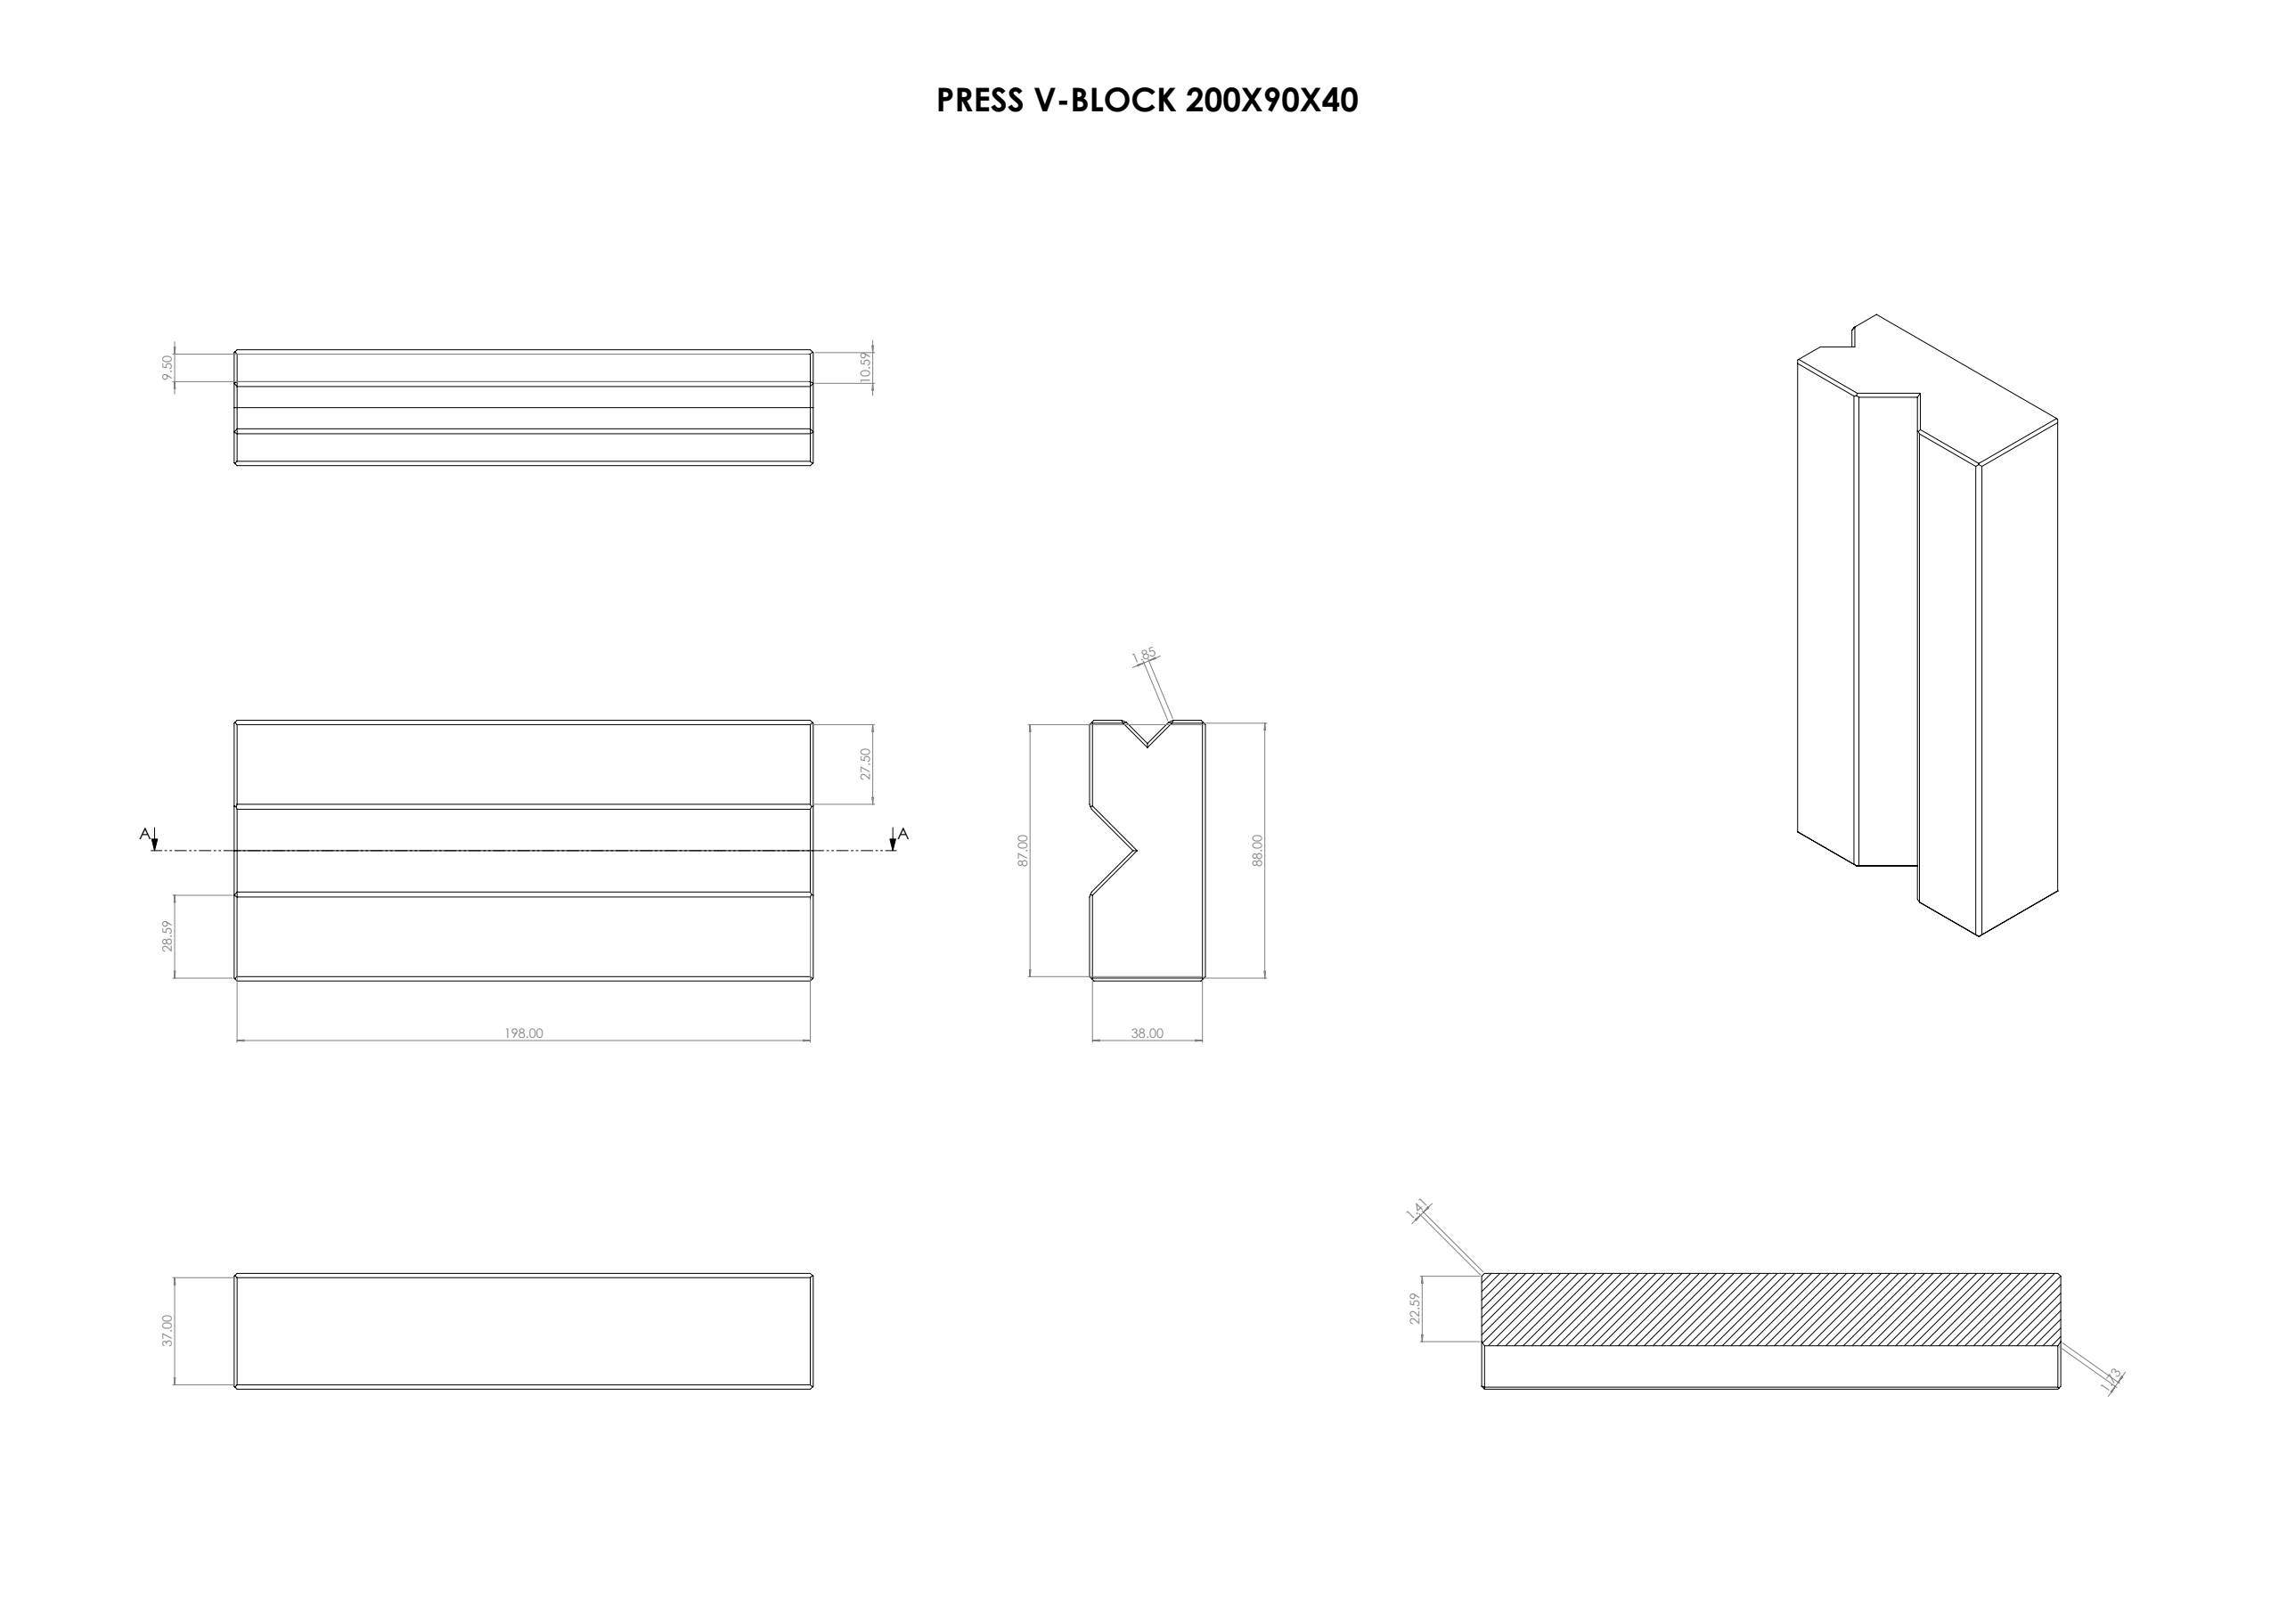
ISO-10303-21;
HEADER;
/* Generated by software containing ST-Developer
 * from STEP Tools, Inc. (www.steptools.com) 
 */

FILE_DESCRIPTION(
/* description */ (''),
/* implementation_level */ '2;1');

FILE_NAME(
/* name */ '16_Press_V-Block_200x90x40.step',
/* time_stamp */ '2026-10-20T10:03:03-07:00',
/* author */ (''),
/* organization */ (''),
/* preprocessor_version */ 'ST-DEVELOPER v20.2',
/* originating_system */ 'Autodesk Translation Framework v15.15.0.0',
/* authorisation */ '');

FILE_SCHEMA (('AUTOMOTIVE_DESIGN { 1 0 10303 214 3 1 1 }'));
ENDSEC;

DATA;
#10=MECHANICAL_DESIGN_GEOMETRIC_PRESENTATION_REPRESENTATION('',(#538),#71492);
#395=SHAPE_REPRESENTATION_RELATIONSHIP('SRR','None',#71616,#414);
#414=ADVANCED_BREP_SHAPE_REPRESENTATION('',(#433),#71486);
#433=MANIFOLD_SOLID_BREP('V-block',#28472);
#538=STYLED_ITEM('',(#71866),#433);
#4118=FACE_OUTER_BOUND('',#5800,.T.);
#4119=FACE_OUTER_BOUND('',#5801,.T.);
#4120=FACE_OUTER_BOUND('',#5802,.T.);
#4121=FACE_OUTER_BOUND('',#5803,.T.);
#4122=FACE_OUTER_BOUND('',#5804,.T.);
#4123=FACE_OUTER_BOUND('',#5805,.T.);
#4124=FACE_OUTER_BOUND('',#5806,.T.);
#4125=FACE_OUTER_BOUND('',#5807,.T.);
#4126=FACE_OUTER_BOUND('',#5808,.T.);
#4127=FACE_OUTER_BOUND('',#5809,.T.);
#4128=FACE_OUTER_BOUND('',#5810,.T.);
#4129=FACE_OUTER_BOUND('',#5811,.T.);
#4130=FACE_OUTER_BOUND('',#5812,.T.);
#4131=FACE_OUTER_BOUND('',#5813,.T.);
#4132=FACE_OUTER_BOUND('',#5814,.T.);
#4133=FACE_OUTER_BOUND('',#5815,.T.);
#4134=FACE_OUTER_BOUND('',#5816,.T.);
#4135=FACE_OUTER_BOUND('',#5817,.T.);
#4136=FACE_OUTER_BOUND('',#5818,.T.);
#4137=FACE_OUTER_BOUND('',#5819,.T.);
#4138=FACE_OUTER_BOUND('',#5820,.T.);
#4139=FACE_OUTER_BOUND('',#5821,.T.);
#4140=FACE_OUTER_BOUND('',#5822,.T.);
#4141=FACE_OUTER_BOUND('',#5823,.T.);
#4142=FACE_OUTER_BOUND('',#5824,.T.);
#4143=FACE_OUTER_BOUND('',#5825,.T.);
#4144=FACE_OUTER_BOUND('',#5826,.T.);
#4145=FACE_OUTER_BOUND('',#5827,.T.);
#4146=FACE_OUTER_BOUND('',#5828,.T.);
#4147=FACE_OUTER_BOUND('',#5829,.T.);
#4148=FACE_OUTER_BOUND('',#5830,.T.);
#4149=FACE_OUTER_BOUND('',#5831,.T.);
#4150=FACE_OUTER_BOUND('',#5832,.T.);
#4151=FACE_OUTER_BOUND('',#5833,.T.);
#4152=FACE_OUTER_BOUND('',#5834,.T.);
#4153=FACE_OUTER_BOUND('',#5835,.T.);
#4154=FACE_OUTER_BOUND('',#5836,.T.);
#4155=FACE_OUTER_BOUND('',#5837,.T.);
#4156=FACE_OUTER_BOUND('',#5838,.T.);
#4157=FACE_OUTER_BOUND('',#5839,.T.);
#4158=FACE_OUTER_BOUND('',#5840,.T.);
#4159=FACE_OUTER_BOUND('',#5841,.T.);
#4160=FACE_OUTER_BOUND('',#5842,.T.);
#4161=FACE_OUTER_BOUND('',#5843,.T.);
#4162=FACE_OUTER_BOUND('',#5844,.T.);
#5800=EDGE_LOOP('',(#23869,#23870,#23871,#23872,#23873,#23874));
#5801=EDGE_LOOP('',(#23875,#23876,#23877,#23878));
#5802=EDGE_LOOP('',(#23879,#23880,#23881,#23882,#23883,#23884));
#5803=EDGE_LOOP('',(#23885,#23886,#23887,#23888,#23889,#23890));
#5804=EDGE_LOOP('',(#23891,#23892,#23893,#23894,#23895,#23896,#23897,#23898,
#23899,#23900));
#5805=EDGE_LOOP('',(#23901,#23902,#23903,#23904));
#5806=EDGE_LOOP('',(#23905,#23906,#23907,#23908,#23909));
#5807=EDGE_LOOP('',(#23910,#23911,#23912,#23913,#23914,#23915));
#5808=EDGE_LOOP('',(#23916,#23917,#23918,#23919,#23920));
#5809=EDGE_LOOP('',(#23921,#23922,#23923,#23924,#23925,#23926));
#5810=EDGE_LOOP('',(#23927,#23928,#23929,#23930));
#5811=EDGE_LOOP('',(#23931,#23932,#23933,#23934,#23935,#23936));
#5812=EDGE_LOOP('',(#23937,#23938,#23939,#23940,#23941));
#5813=EDGE_LOOP('',(#23942,#23943,#23944,#23945));
#5814=EDGE_LOOP('',(#23946,#23947,#23948,#23949,#23950,#23951));
#5815=EDGE_LOOP('',(#23952,#23953,#23954,#23955,#23956,#23957));
#5816=EDGE_LOOP('',(#23958,#23959,#23960,#23961,#23962));
#5817=EDGE_LOOP('',(#23963,#23964,#23965));
#5818=EDGE_LOOP('',(#23966,#23967,#23968,#23969));
#5819=EDGE_LOOP('',(#23970,#23971,#23972,#23973,#23974));
#5820=EDGE_LOOP('',(#23975,#23976,#23977,#23978,#23979));
#5821=EDGE_LOOP('',(#23980,#23981,#23982,#23983));
#5822=EDGE_LOOP('',(#23984,#23985,#23986,#23987,#23988,#23989));
#5823=EDGE_LOOP('',(#23990,#23991,#23992,#23993,#23994,#23995));
#5824=EDGE_LOOP('',(#23996,#23997,#23998,#23999,#24000,#24001));
#5825=EDGE_LOOP('',(#24002,#24003,#24004,#24005,#24006));
#5826=EDGE_LOOP('',(#24007,#24008,#24009));
#5827=EDGE_LOOP('',(#24010,#24011,#24012,#24013,#24014));
#5828=EDGE_LOOP('',(#24015,#24016,#24017));
#5829=EDGE_LOOP('',(#24018,#24019,#24020,#24021));
#5830=EDGE_LOOP('',(#24022,#24023,#24024));
#5831=EDGE_LOOP('',(#24025,#24026,#24027,#24028));
#5832=EDGE_LOOP('',(#24029,#24030,#24031,#24032,#24033));
#5833=EDGE_LOOP('',(#24034,#24035,#24036));
#5834=EDGE_LOOP('',(#24037,#24038,#24039,#24040));
#5835=EDGE_LOOP('',(#24041,#24042,#24043,#24044));
#5836=EDGE_LOOP('',(#24045,#24046,#24047,#24048));
#5837=EDGE_LOOP('',(#24049,#24050,#24051,#24052));
#5838=EDGE_LOOP('',(#24053,#24054,#24055,#24056));
#5839=EDGE_LOOP('',(#24057,#24058,#24059,#24060,#24061,#24062,#24063,#24064,
#24065,#24066));
#5840=EDGE_LOOP('',(#24067,#24068,#24069,#24070));
#5841=EDGE_LOOP('',(#24071,#24072,#24073,#24074));
#5842=EDGE_LOOP('',(#24075,#24076,#24077,#24078));
#5843=EDGE_LOOP('',(#24079,#24080,#24081,#24082,#24083,#24084));
#5844=EDGE_LOOP('',(#24085,#24086,#24087,#24088));
#8268=LINE('',#58858,#10756);
#8269=LINE('',#58860,#10757);
#8270=LINE('',#58862,#10758);
#8271=LINE('',#58864,#10759);
#8272=LINE('',#58866,#10760);
#8273=LINE('',#58867,#10761);
#8274=LINE('',#58870,#10762);
#8275=LINE('',#58872,#10763);
#8276=LINE('',#58873,#10764);
#8277=LINE('',#58876,#10765);
#8278=LINE('',#58878,#10766);
#8279=LINE('',#58880,#10767);
#8280=LINE('',#58881,#10768);
#8281=LINE('',#58884,#10769);
#8282=LINE('',#58886,#10770);
#8283=LINE('',#58888,#10771);
#8284=LINE('',#58889,#10772);
#8285=LINE('',#58892,#10773);
#8286=LINE('',#58894,#10774);
#8287=LINE('',#58896,#10775);
#8288=LINE('',#58898,#10776);
#8289=LINE('',#58900,#10777);
#8290=LINE('',#58902,#10778);
#8291=LINE('',#58904,#10779);
#8292=LINE('',#58905,#10780);
#8293=LINE('',#58908,#10781);
#8294=LINE('',#58909,#10782);
#8295=LINE('',#58912,#10783);
#8296=LINE('',#58914,#10784);
#8297=LINE('',#58916,#10785);
#8298=LINE('',#58917,#10786);
#8299=LINE('',#58920,#10787);
#8300=LINE('',#58922,#10788);
#8301=LINE('',#58923,#10789);
#8302=LINE('',#58926,#10790);
#8303=LINE('',#58928,#10791);
#8304=LINE('',#58929,#10792);
#8305=LINE('',#58933,#10793);
#8306=LINE('',#58935,#10794);
#8307=LINE('',#58937,#10795);
#8308=LINE('',#58939,#10796);
#8309=LINE('',#58941,#10797);
#8310=LINE('',#58942,#10798);
#8311=LINE('',#58945,#10799);
#8312=LINE('',#58947,#10800);
#8313=LINE('',#58948,#10801);
#8314=LINE('',#58950,#10802);
#8315=LINE('',#58952,#10803);
#8316=LINE('',#58953,#10804);
#8317=LINE('',#58955,#10805);
#8318=LINE('',#58958,#10806);
#8319=LINE('',#58959,#10807);
#8320=LINE('',#58962,#10808);
#8321=LINE('',#58964,#10809);
#8322=LINE('',#58966,#10810);
#8323=LINE('',#58967,#10811);
#8324=LINE('',#58970,#10812);
#8325=LINE('',#58972,#10813);
#8326=LINE('',#58973,#10814);
#8327=LINE('',#58976,#10815);
#8328=LINE('',#58977,#10816);
#8329=LINE('',#58980,#10817);
#8330=LINE('',#58981,#10818);
#8331=LINE('',#58983,#10819);
#8332=LINE('',#58984,#10820);
#8333=LINE('',#58988,#10821);
#8334=LINE('',#58989,#10822);
#8335=LINE('',#58991,#10823);
#8336=LINE('',#58992,#10824);
#8337=LINE('',#58995,#10825);
#8338=LINE('',#58997,#10826);
#8339=LINE('',#58998,#10827);
#8340=LINE('',#59002,#10828);
#8341=LINE('',#59003,#10829);
#8342=LINE('',#59004,#10830);
#8343=LINE('',#59007,#10831);
#8344=LINE('',#59009,#10832);
#8345=LINE('',#59010,#10833);
#8346=LINE('',#59013,#10834);
#8347=LINE('',#59015,#10835);
#8348=LINE('',#59016,#10836);
#8349=LINE('',#59019,#10837);
#8350=LINE('',#59021,#10838);
#8351=LINE('',#59022,#10839);
#8352=LINE('',#59026,#10840);
#8353=LINE('',#59027,#10841);
#8354=LINE('',#59028,#10842);
#8355=LINE('',#59030,#10843);
#8356=LINE('',#59033,#10844);
#8357=LINE('',#59034,#10845);
#8358=LINE('',#59036,#10846);
#8359=LINE('',#59037,#10847);
#8360=LINE('',#59041,#10848);
#8361=LINE('',#59042,#10849);
#8362=LINE('',#59043,#10850);
#8363=LINE('',#59046,#10851);
#8364=LINE('',#59047,#10852);
#8365=LINE('',#59049,#10853);
#8366=LINE('',#59052,#10854);
#8367=LINE('',#59053,#10855);
#8368=LINE('',#59056,#10856);
#8369=LINE('',#59058,#10857);
#8370=LINE('',#59059,#10858);
#8371=LINE('',#59061,#10859);
#8372=LINE('',#59062,#10860);
#8373=LINE('',#59064,#10861);
#8374=LINE('',#59065,#10862);
#8375=LINE('',#59067,#10863);
#8376=LINE('',#59071,#10864);
#8377=LINE('',#59075,#10865);
#10756=VECTOR('',#35925,1.);
#10757=VECTOR('',#35926,1.);
#10758=VECTOR('',#35927,1.);
#10759=VECTOR('',#35928,1.);
#10760=VECTOR('',#35929,1.);
#10761=VECTOR('',#35930,1.);
#10762=VECTOR('',#35933,1.);
#10763=VECTOR('',#35934,1.);
#10764=VECTOR('',#35935,1.);
#10765=VECTOR('',#35938,1.);
#10766=VECTOR('',#35939,1.);
#10767=VECTOR('',#35940,1.);
#10768=VECTOR('',#35941,1.);
#10769=VECTOR('',#35944,1.);
#10770=VECTOR('',#35945,1.);
#10771=VECTOR('',#35946,1.);
#10772=VECTOR('',#35947,1.);
#10773=VECTOR('',#35950,1.);
#10774=VECTOR('',#35951,1.);
#10775=VECTOR('',#35952,1.);
#10776=VECTOR('',#35953,1.);
#10777=VECTOR('',#35954,1.);
#10778=VECTOR('',#35955,1.);
#10779=VECTOR('',#35956,1.);
#10780=VECTOR('',#35957,1.);
#10781=VECTOR('',#35960,1.);
#10782=VECTOR('',#35961,1.);
#10783=VECTOR('',#35964,1.);
#10784=VECTOR('',#35965,1.);
#10785=VECTOR('',#35966,1.);
#10786=VECTOR('',#35967,1.);
#10787=VECTOR('',#35970,1.);
#10788=VECTOR('',#35971,1.);
#10789=VECTOR('',#35972,1.);
#10790=VECTOR('',#35975,1.);
#10791=VECTOR('',#35976,1.);
#10792=VECTOR('',#35977,1.);
#10793=VECTOR('',#35980,1.);
#10794=VECTOR('',#35981,1.);
#10795=VECTOR('',#35982,1.);
#10796=VECTOR('',#35983,1.);
#10797=VECTOR('',#35984,1.);
#10798=VECTOR('',#35985,1.);
#10799=VECTOR('',#35988,1.);
#10800=VECTOR('',#35989,1.);
#10801=VECTOR('',#35990,1.);
#10802=VECTOR('',#35993,1.);
#10803=VECTOR('',#35994,1.);
#10804=VECTOR('',#35995,1.);
#10805=VECTOR('',#35998,1.);
#10806=VECTOR('',#36001,1.);
#10807=VECTOR('',#36002,1.);
#10808=VECTOR('',#36005,1.);
#10809=VECTOR('',#36006,1.);
#10810=VECTOR('',#36007,1.);
#10811=VECTOR('',#36008,1.);
#10812=VECTOR('',#36011,1.);
#10813=VECTOR('',#36012,1.);
#10814=VECTOR('',#36013,1.);
#10815=VECTOR('',#36016,1.);
#10816=VECTOR('',#36017,1.);
#10817=VECTOR('',#36020,1.);
#10818=VECTOR('',#36021,1.);
#10819=VECTOR('',#36024,1.);
#10820=VECTOR('',#36025,1.);
#10821=VECTOR('',#36028,1.);
#10822=VECTOR('',#36029,1.);
#10823=VECTOR('',#36030,1.);
#10824=VECTOR('',#36031,1.);
#10825=VECTOR('',#36034,1.);
#10826=VECTOR('',#36035,1.);
#10827=VECTOR('',#36036,1.);
#10828=VECTOR('',#36041,1.);
#10829=VECTOR('',#36042,1.);
#10830=VECTOR('',#36043,1.);
#10831=VECTOR('',#36046,1.);
#10832=VECTOR('',#36047,1.);
#10833=VECTOR('',#36048,1.);
#10834=VECTOR('',#36051,1.);
#10835=VECTOR('',#36052,1.);
#10836=VECTOR('',#36053,1.);
#10837=VECTOR('',#36056,1.);
#10838=VECTOR('',#36057,1.);
#10839=VECTOR('',#36058,1.);
#10840=VECTOR('',#36061,1.);
#10841=VECTOR('',#36062,1.);
#10842=VECTOR('',#36063,1.);
#10843=VECTOR('',#36066,1.);
#10844=VECTOR('',#36069,1.);
#10845=VECTOR('',#36070,1.);
#10846=VECTOR('',#36073,1.);
#10847=VECTOR('',#36074,1.);
#10848=VECTOR('',#36077,1.);
#10849=VECTOR('',#36078,1.);
#10850=VECTOR('',#36079,1.);
#10851=VECTOR('',#36082,1.);
#10852=VECTOR('',#36083,1.);
#10853=VECTOR('',#36086,1.);
#10854=VECTOR('',#36089,1.);
#10855=VECTOR('',#36090,1.);
#10856=VECTOR('',#36093,1.);
#10857=VECTOR('',#36094,1.);
#10858=VECTOR('',#36095,1.);
#10859=VECTOR('',#36098,1.);
#10860=VECTOR('',#36099,1.);
#10861=VECTOR('',#36102,1.);
#10862=VECTOR('',#36103,1.);
#10863=VECTOR('',#36106,1.);
#10864=VECTOR('',#36113,1.);
#10865=VECTOR('',#36120,1.);
#13146=VERTEX_POINT('',#58856);
#13147=VERTEX_POINT('',#58857);
#13148=VERTEX_POINT('',#58859);
#13149=VERTEX_POINT('',#58861);
#13150=VERTEX_POINT('',#58863);
#13151=VERTEX_POINT('',#58865);
#13152=VERTEX_POINT('',#58869);
#13153=VERTEX_POINT('',#58871);
#13154=VERTEX_POINT('',#58875);
#13155=VERTEX_POINT('',#58877);
#13156=VERTEX_POINT('',#58879);
#13157=VERTEX_POINT('',#58883);
#13158=VERTEX_POINT('',#58885);
#13159=VERTEX_POINT('',#58887);
#13160=VERTEX_POINT('',#58891);
#13161=VERTEX_POINT('',#58893);
#13162=VERTEX_POINT('',#58895);
#13163=VERTEX_POINT('',#58897);
#13164=VERTEX_POINT('',#58899);
#13165=VERTEX_POINT('',#58901);
#13166=VERTEX_POINT('',#58903);
#13167=VERTEX_POINT('',#58907);
#13168=VERTEX_POINT('',#58911);
#13169=VERTEX_POINT('',#58913);
#13170=VERTEX_POINT('',#58915);
#13171=VERTEX_POINT('',#58919);
#13172=VERTEX_POINT('',#58921);
#13173=VERTEX_POINT('',#58925);
#13174=VERTEX_POINT('',#58927);
#13175=VERTEX_POINT('',#58931);
#13176=VERTEX_POINT('',#58932);
#13177=VERTEX_POINT('',#58934);
#13178=VERTEX_POINT('',#58936);
#13179=VERTEX_POINT('',#58938);
#13180=VERTEX_POINT('',#58940);
#13181=VERTEX_POINT('',#58944);
#13182=VERTEX_POINT('',#58946);
#13183=VERTEX_POINT('',#58951);
#13184=VERTEX_POINT('',#58957);
#13185=VERTEX_POINT('',#58961);
#13186=VERTEX_POINT('',#58963);
#13187=VERTEX_POINT('',#58965);
#13188=VERTEX_POINT('',#58969);
#13189=VERTEX_POINT('',#58971);
#13190=VERTEX_POINT('',#58975);
#13191=VERTEX_POINT('',#58979);
#13192=VERTEX_POINT('',#58986);
#13193=VERTEX_POINT('',#58987);
#13194=VERTEX_POINT('',#58990);
#13195=VERTEX_POINT('',#58994);
#13196=VERTEX_POINT('',#58996);
#13197=VERTEX_POINT('',#59001);
#13198=VERTEX_POINT('',#59006);
#13199=VERTEX_POINT('',#59008);
#13200=VERTEX_POINT('',#59012);
#13201=VERTEX_POINT('',#59014);
#13202=VERTEX_POINT('',#59018);
#13203=VERTEX_POINT('',#59020);
#13204=VERTEX_POINT('',#59024);
#13205=VERTEX_POINT('',#59025);
#13206=VERTEX_POINT('',#59032);
#13207=VERTEX_POINT('',#59039);
#13208=VERTEX_POINT('',#59040);
#13209=VERTEX_POINT('',#59045);
#13210=VERTEX_POINT('',#59051);
#13211=VERTEX_POINT('',#59055);
#13212=VERTEX_POINT('',#59057);
#16818=EDGE_CURVE('',#13146,#13147,#8268,.T.);
#16819=EDGE_CURVE('',#13147,#13148,#8269,.T.);
#16820=EDGE_CURVE('',#13148,#13149,#8270,.T.);
#16821=EDGE_CURVE('',#13149,#13150,#8271,.T.);
#16822=EDGE_CURVE('',#13150,#13151,#8272,.T.);
#16823=EDGE_CURVE('',#13151,#13146,#8273,.T.);
#16824=EDGE_CURVE('',#13152,#13150,#8274,.T.);
#16825=EDGE_CURVE('',#13153,#13152,#8275,.T.);
#16826=EDGE_CURVE('',#13151,#13153,#8276,.T.);
#16827=EDGE_CURVE('',#13154,#13149,#8277,.T.);
#16828=EDGE_CURVE('',#13154,#13155,#8278,.T.);
#16829=EDGE_CURVE('',#13156,#13155,#8279,.T.);
#16830=EDGE_CURVE('',#13152,#13156,#8280,.T.);
#16831=EDGE_CURVE('',#13148,#13157,#8281,.T.);
#16832=EDGE_CURVE('',#13157,#13158,#8282,.T.);
#16833=EDGE_CURVE('',#13158,#13159,#8283,.T.);
#16834=EDGE_CURVE('',#13159,#13154,#8284,.T.);
#16835=EDGE_CURVE('',#13160,#13147,#8285,.T.);
#16836=EDGE_CURVE('',#13161,#13160,#8286,.T.);
#16837=EDGE_CURVE('',#13162,#13161,#8287,.T.);
#16838=EDGE_CURVE('',#13163,#13162,#8288,.T.);
#16839=EDGE_CURVE('',#13164,#13163,#8289,.T.);
#16840=EDGE_CURVE('',#13165,#13164,#8290,.T.);
#16841=EDGE_CURVE('',#13166,#13165,#8291,.T.);
#16842=EDGE_CURVE('',#13157,#13166,#8292,.T.);
#16843=EDGE_CURVE('',#13167,#13159,#8293,.T.);
#16844=EDGE_CURVE('',#13155,#13167,#8294,.T.);
#16845=EDGE_CURVE('',#13168,#13166,#8295,.T.);
#16846=EDGE_CURVE('',#13165,#13169,#8296,.F.);
#16847=EDGE_CURVE('',#13169,#13170,#8297,.T.);
#16848=EDGE_CURVE('',#13170,#13168,#8298,.T.);
#16849=EDGE_CURVE('',#13171,#13168,#8299,.T.);
#16850=EDGE_CURVE('',#13171,#13172,#8300,.T.);
#16851=EDGE_CURVE('',#13172,#13158,#8301,.T.);
#16852=EDGE_CURVE('',#13170,#13173,#8302,.T.);
#16853=EDGE_CURVE('',#13173,#13174,#8303,.T.);
#16854=EDGE_CURVE('',#13174,#13171,#8304,.T.);
#16855=EDGE_CURVE('',#13175,#13176,#8305,.T.);
#16856=EDGE_CURVE('',#13176,#13177,#8306,.T.);
#16857=EDGE_CURVE('',#13177,#13178,#8307,.T.);
#16858=EDGE_CURVE('',#13178,#13179,#8308,.T.);
#16859=EDGE_CURVE('',#13179,#13180,#8309,.T.);
#16860=EDGE_CURVE('',#13180,#13175,#8310,.T.);
#16861=EDGE_CURVE('',#13181,#13176,#8311,.T.);
#16862=EDGE_CURVE('',#13182,#13181,#8312,.T.);
#16863=EDGE_CURVE('',#13177,#13182,#8313,.T.);
#16864=EDGE_CURVE('',#13164,#13175,#8314,.T.);
#16865=EDGE_CURVE('',#13163,#13183,#8315,.T.);
#16866=EDGE_CURVE('',#13183,#13181,#8316,.T.);
#16867=EDGE_CURVE('',#13180,#13169,#8317,.T.);
#16868=EDGE_CURVE('',#13184,#13179,#8318,.T.);
#16869=EDGE_CURVE('',#13184,#13169,#8319,.T.);
#16870=EDGE_CURVE('',#13185,#13183,#8320,.T.);
#16871=EDGE_CURVE('',#13185,#13186,#8321,.T.);
#16872=EDGE_CURVE('',#13187,#13186,#8322,.T.);
#16873=EDGE_CURVE('',#13182,#13187,#8323,.T.);
#16874=EDGE_CURVE('',#13187,#13188,#8324,.T.);
#16875=EDGE_CURVE('',#13188,#13189,#8325,.T.);
#16876=EDGE_CURVE('',#13189,#13178,#8326,.T.);
#16877=EDGE_CURVE('',#13189,#13190,#8327,.T.);
#16878=EDGE_CURVE('',#13190,#13184,#8328,.T.);
#16879=EDGE_CURVE('',#13191,#13173,#8329,.T.);
#16880=EDGE_CURVE('',#13174,#13191,#8330,.T.);
#16881=EDGE_CURVE('',#13190,#13191,#8331,.T.);
#16882=EDGE_CURVE('',#13173,#13184,#8332,.T.);
#16883=EDGE_CURVE('',#13192,#13193,#8333,.T.);
#16884=EDGE_CURVE('',#13193,#13174,#8334,.T.);
#16885=EDGE_CURVE('',#13191,#13194,#8335,.T.);
#16886=EDGE_CURVE('',#13194,#13192,#8336,.T.);
#16887=EDGE_CURVE('',#13186,#13195,#8337,.T.);
#16888=EDGE_CURVE('',#13195,#13196,#8338,.T.);
#16889=EDGE_CURVE('',#13196,#13188,#8339,.T.);
#16890=EDGE_CURVE('',#13194,#13197,#8340,.T.);
#16891=EDGE_CURVE('',#13197,#13156,#8341,.T.);
#16892=EDGE_CURVE('',#13167,#13192,#8342,.T.);
#16893=EDGE_CURVE('',#13197,#13198,#8343,.T.);
#16894=EDGE_CURVE('',#13198,#13199,#8344,.T.);
#16895=EDGE_CURVE('',#13199,#13153,#8345,.T.);
#16896=EDGE_CURVE('',#13200,#13199,#8346,.T.);
#16897=EDGE_CURVE('',#13200,#13201,#8347,.T.);
#16898=EDGE_CURVE('',#13146,#13201,#8348,.T.);
#16899=EDGE_CURVE('',#13198,#13202,#8349,.T.);
#16900=EDGE_CURVE('',#13202,#13203,#8350,.T.);
#16901=EDGE_CURVE('',#13203,#13200,#8351,.T.);
#16902=EDGE_CURVE('',#13204,#13205,#8352,.T.);
#16903=EDGE_CURVE('',#13162,#13204,#8353,.T.);
#16904=EDGE_CURVE('',#13205,#13162,#8354,.T.);
#16905=EDGE_CURVE('',#13204,#13185,#8355,.T.);
#16906=EDGE_CURVE('',#13206,#13195,#8356,.T.);
#16907=EDGE_CURVE('',#13196,#13206,#8357,.T.);
#16908=EDGE_CURVE('',#13195,#13204,#8358,.T.);
#16909=EDGE_CURVE('',#13205,#13206,#8359,.T.);
#16910=EDGE_CURVE('',#13207,#13208,#8360,.T.);
#16911=EDGE_CURVE('',#13160,#13207,#8361,.T.);
#16912=EDGE_CURVE('',#13208,#13160,#8362,.T.);
#16913=EDGE_CURVE('',#13207,#13209,#8363,.T.);
#16914=EDGE_CURVE('',#13209,#13161,#8364,.T.);
#16915=EDGE_CURVE('',#13201,#13208,#8365,.T.);
#16916=EDGE_CURVE('',#13203,#13210,#8366,.T.);
#16917=EDGE_CURVE('',#13210,#13202,#8367,.T.);
#16918=EDGE_CURVE('',#13211,#13210,#8368,.T.);
#16919=EDGE_CURVE('',#13202,#13212,#8369,.T.);
#16920=EDGE_CURVE('',#13212,#13211,#8370,.T.);
#16921=EDGE_CURVE('',#13208,#13203,#8371,.T.);
#16922=EDGE_CURVE('',#13210,#13207,#8372,.T.);
#16923=EDGE_CURVE('',#13212,#13196,#8373,.T.);
#16924=EDGE_CURVE('',#13206,#13211,#8374,.T.);
#16925=EDGE_CURVE('',#13209,#13205,#8375,.T.);
#16926=EDGE_CURVE('',#13211,#13209,#8376,.T.);
#16927=EDGE_CURVE('',#13172,#13193,#8377,.T.);
#23869=ORIENTED_EDGE('',*,*,#16818,.T.);
#23870=ORIENTED_EDGE('',*,*,#16819,.T.);
#23871=ORIENTED_EDGE('',*,*,#16820,.T.);
#23872=ORIENTED_EDGE('',*,*,#16821,.T.);
#23873=ORIENTED_EDGE('',*,*,#16822,.T.);
#23874=ORIENTED_EDGE('',*,*,#16823,.T.);
#23875=ORIENTED_EDGE('',*,*,#16822,.F.);
#23876=ORIENTED_EDGE('',*,*,#16824,.F.);
#23877=ORIENTED_EDGE('',*,*,#16825,.F.);
#23878=ORIENTED_EDGE('',*,*,#16826,.F.);
#23879=ORIENTED_EDGE('',*,*,#16821,.F.);
#23880=ORIENTED_EDGE('',*,*,#16827,.F.);
#23881=ORIENTED_EDGE('',*,*,#16828,.T.);
#23882=ORIENTED_EDGE('',*,*,#16829,.F.);
#23883=ORIENTED_EDGE('',*,*,#16830,.F.);
#23884=ORIENTED_EDGE('',*,*,#16824,.T.);
#23885=ORIENTED_EDGE('',*,*,#16820,.F.);
#23886=ORIENTED_EDGE('',*,*,#16831,.T.);
#23887=ORIENTED_EDGE('',*,*,#16832,.T.);
#23888=ORIENTED_EDGE('',*,*,#16833,.T.);
#23889=ORIENTED_EDGE('',*,*,#16834,.T.);
#23890=ORIENTED_EDGE('',*,*,#16827,.T.);
#23891=ORIENTED_EDGE('',*,*,#16819,.F.);
#23892=ORIENTED_EDGE('',*,*,#16835,.F.);
#23893=ORIENTED_EDGE('',*,*,#16836,.F.);
#23894=ORIENTED_EDGE('',*,*,#16837,.F.);
#23895=ORIENTED_EDGE('',*,*,#16838,.F.);
#23896=ORIENTED_EDGE('',*,*,#16839,.F.);
#23897=ORIENTED_EDGE('',*,*,#16840,.F.);
#23898=ORIENTED_EDGE('',*,*,#16841,.F.);
#23899=ORIENTED_EDGE('',*,*,#16842,.F.);
#23900=ORIENTED_EDGE('',*,*,#16831,.F.);
#23901=ORIENTED_EDGE('',*,*,#16834,.F.);
#23902=ORIENTED_EDGE('',*,*,#16843,.F.);
#23903=ORIENTED_EDGE('',*,*,#16844,.F.);
#23904=ORIENTED_EDGE('',*,*,#16828,.F.);
#23905=ORIENTED_EDGE('',*,*,#16845,.T.);
#23906=ORIENTED_EDGE('',*,*,#16841,.T.);
#23907=ORIENTED_EDGE('',*,*,#16846,.T.);
#23908=ORIENTED_EDGE('',*,*,#16847,.T.);
#23909=ORIENTED_EDGE('',*,*,#16848,.T.);
#23910=ORIENTED_EDGE('',*,*,#16832,.F.);
#23911=ORIENTED_EDGE('',*,*,#16842,.T.);
#23912=ORIENTED_EDGE('',*,*,#16845,.F.);
#23913=ORIENTED_EDGE('',*,*,#16849,.F.);
#23914=ORIENTED_EDGE('',*,*,#16850,.T.);
#23915=ORIENTED_EDGE('',*,*,#16851,.T.);
#23916=ORIENTED_EDGE('',*,*,#16848,.F.);
#23917=ORIENTED_EDGE('',*,*,#16852,.T.);
#23918=ORIENTED_EDGE('',*,*,#16853,.T.);
#23919=ORIENTED_EDGE('',*,*,#16854,.T.);
#23920=ORIENTED_EDGE('',*,*,#16849,.T.);
#23921=ORIENTED_EDGE('',*,*,#16855,.T.);
#23922=ORIENTED_EDGE('',*,*,#16856,.T.);
#23923=ORIENTED_EDGE('',*,*,#16857,.T.);
#23924=ORIENTED_EDGE('',*,*,#16858,.T.);
#23925=ORIENTED_EDGE('',*,*,#16859,.T.);
#23926=ORIENTED_EDGE('',*,*,#16860,.T.);
#23927=ORIENTED_EDGE('',*,*,#16856,.F.);
#23928=ORIENTED_EDGE('',*,*,#16861,.F.);
#23929=ORIENTED_EDGE('',*,*,#16862,.F.);
#23930=ORIENTED_EDGE('',*,*,#16863,.F.);
#23931=ORIENTED_EDGE('',*,*,#16855,.F.);
#23932=ORIENTED_EDGE('',*,*,#16864,.F.);
#23933=ORIENTED_EDGE('',*,*,#16839,.T.);
#23934=ORIENTED_EDGE('',*,*,#16865,.T.);
#23935=ORIENTED_EDGE('',*,*,#16866,.T.);
#23936=ORIENTED_EDGE('',*,*,#16861,.T.);
#23937=ORIENTED_EDGE('',*,*,#16860,.F.);
#23938=ORIENTED_EDGE('',*,*,#16867,.T.);
#23939=ORIENTED_EDGE('',*,*,#16846,.F.);
#23940=ORIENTED_EDGE('',*,*,#16840,.T.);
#23941=ORIENTED_EDGE('',*,*,#16864,.T.);
#23942=ORIENTED_EDGE('',*,*,#16859,.F.);
#23943=ORIENTED_EDGE('',*,*,#16868,.F.);
#23944=ORIENTED_EDGE('',*,*,#16869,.T.);
#23945=ORIENTED_EDGE('',*,*,#16867,.F.);
#23946=ORIENTED_EDGE('',*,*,#16866,.F.);
#23947=ORIENTED_EDGE('',*,*,#16870,.F.);
#23948=ORIENTED_EDGE('',*,*,#16871,.T.);
#23949=ORIENTED_EDGE('',*,*,#16872,.F.);
#23950=ORIENTED_EDGE('',*,*,#16873,.F.);
#23951=ORIENTED_EDGE('',*,*,#16862,.T.);
#23952=ORIENTED_EDGE('',*,*,#16857,.F.);
#23953=ORIENTED_EDGE('',*,*,#16863,.T.);
#23954=ORIENTED_EDGE('',*,*,#16873,.T.);
#23955=ORIENTED_EDGE('',*,*,#16874,.T.);
#23956=ORIENTED_EDGE('',*,*,#16875,.T.);
#23957=ORIENTED_EDGE('',*,*,#16876,.T.);
#23958=ORIENTED_EDGE('',*,*,#16858,.F.);
#23959=ORIENTED_EDGE('',*,*,#16876,.F.);
#23960=ORIENTED_EDGE('',*,*,#16877,.T.);
#23961=ORIENTED_EDGE('',*,*,#16878,.T.);
#23962=ORIENTED_EDGE('',*,*,#16868,.T.);
#23963=ORIENTED_EDGE('',*,*,#16853,.F.);
#23964=ORIENTED_EDGE('',*,*,#16879,.F.);
#23965=ORIENTED_EDGE('',*,*,#16880,.F.);
#23966=ORIENTED_EDGE('',*,*,#16881,.T.);
#23967=ORIENTED_EDGE('',*,*,#16879,.T.);
#23968=ORIENTED_EDGE('',*,*,#16882,.T.);
#23969=ORIENTED_EDGE('',*,*,#16878,.F.);
#23970=ORIENTED_EDGE('',*,*,#16883,.T.);
#23971=ORIENTED_EDGE('',*,*,#16884,.T.);
#23972=ORIENTED_EDGE('',*,*,#16880,.T.);
#23973=ORIENTED_EDGE('',*,*,#16885,.T.);
#23974=ORIENTED_EDGE('',*,*,#16886,.T.);
#23975=ORIENTED_EDGE('',*,*,#16874,.F.);
#23976=ORIENTED_EDGE('',*,*,#16872,.T.);
#23977=ORIENTED_EDGE('',*,*,#16887,.T.);
#23978=ORIENTED_EDGE('',*,*,#16888,.T.);
#23979=ORIENTED_EDGE('',*,*,#16889,.T.);
#23980=ORIENTED_EDGE('',*,*,#16847,.F.);
#23981=ORIENTED_EDGE('',*,*,#16869,.F.);
#23982=ORIENTED_EDGE('',*,*,#16882,.F.);
#23983=ORIENTED_EDGE('',*,*,#16852,.F.);
#23984=ORIENTED_EDGE('',*,*,#16886,.F.);
#23985=ORIENTED_EDGE('',*,*,#16890,.T.);
#23986=ORIENTED_EDGE('',*,*,#16891,.T.);
#23987=ORIENTED_EDGE('',*,*,#16829,.T.);
#23988=ORIENTED_EDGE('',*,*,#16844,.T.);
#23989=ORIENTED_EDGE('',*,*,#16892,.T.);
#23990=ORIENTED_EDGE('',*,*,#16891,.F.);
#23991=ORIENTED_EDGE('',*,*,#16893,.T.);
#23992=ORIENTED_EDGE('',*,*,#16894,.T.);
#23993=ORIENTED_EDGE('',*,*,#16895,.T.);
#23994=ORIENTED_EDGE('',*,*,#16825,.T.);
#23995=ORIENTED_EDGE('',*,*,#16830,.T.);
#23996=ORIENTED_EDGE('',*,*,#16823,.F.);
#23997=ORIENTED_EDGE('',*,*,#16826,.T.);
#23998=ORIENTED_EDGE('',*,*,#16895,.F.);
#23999=ORIENTED_EDGE('',*,*,#16896,.F.);
#24000=ORIENTED_EDGE('',*,*,#16897,.T.);
#24001=ORIENTED_EDGE('',*,*,#16898,.F.);
#24002=ORIENTED_EDGE('',*,*,#16894,.F.);
#24003=ORIENTED_EDGE('',*,*,#16899,.T.);
#24004=ORIENTED_EDGE('',*,*,#16900,.T.);
#24005=ORIENTED_EDGE('',*,*,#16901,.T.);
#24006=ORIENTED_EDGE('',*,*,#16896,.T.);
#24007=ORIENTED_EDGE('',*,*,#16902,.F.);
#24008=ORIENTED_EDGE('',*,*,#16903,.F.);
#24009=ORIENTED_EDGE('',*,*,#16904,.F.);
#24010=ORIENTED_EDGE('',*,*,#16865,.F.);
#24011=ORIENTED_EDGE('',*,*,#16838,.T.);
#24012=ORIENTED_EDGE('',*,*,#16903,.T.);
#24013=ORIENTED_EDGE('',*,*,#16905,.T.);
#24014=ORIENTED_EDGE('',*,*,#16870,.T.);
#24015=ORIENTED_EDGE('',*,*,#16888,.F.);
#24016=ORIENTED_EDGE('',*,*,#16906,.F.);
#24017=ORIENTED_EDGE('',*,*,#16907,.F.);
#24018=ORIENTED_EDGE('',*,*,#16906,.T.);
#24019=ORIENTED_EDGE('',*,*,#16908,.T.);
#24020=ORIENTED_EDGE('',*,*,#16902,.T.);
#24021=ORIENTED_EDGE('',*,*,#16909,.T.);
#24022=ORIENTED_EDGE('',*,*,#16910,.F.);
#24023=ORIENTED_EDGE('',*,*,#16911,.F.);
#24024=ORIENTED_EDGE('',*,*,#16912,.F.);
#24025=ORIENTED_EDGE('',*,*,#16836,.T.);
#24026=ORIENTED_EDGE('',*,*,#16911,.T.);
#24027=ORIENTED_EDGE('',*,*,#16913,.T.);
#24028=ORIENTED_EDGE('',*,*,#16914,.T.);
#24029=ORIENTED_EDGE('',*,*,#16818,.F.);
#24030=ORIENTED_EDGE('',*,*,#16898,.T.);
#24031=ORIENTED_EDGE('',*,*,#16915,.T.);
#24032=ORIENTED_EDGE('',*,*,#16912,.T.);
#24033=ORIENTED_EDGE('',*,*,#16835,.T.);
#24034=ORIENTED_EDGE('',*,*,#16916,.F.);
#24035=ORIENTED_EDGE('',*,*,#16900,.F.);
#24036=ORIENTED_EDGE('',*,*,#16917,.F.);
#24037=ORIENTED_EDGE('',*,*,#16918,.T.);
#24038=ORIENTED_EDGE('',*,*,#16917,.T.);
#24039=ORIENTED_EDGE('',*,*,#16919,.T.);
#24040=ORIENTED_EDGE('',*,*,#16920,.T.);
#24041=ORIENTED_EDGE('',*,*,#16910,.T.);
#24042=ORIENTED_EDGE('',*,*,#16921,.T.);
#24043=ORIENTED_EDGE('',*,*,#16916,.T.);
#24044=ORIENTED_EDGE('',*,*,#16922,.T.);
#24045=ORIENTED_EDGE('',*,*,#16923,.T.);
#24046=ORIENTED_EDGE('',*,*,#16907,.T.);
#24047=ORIENTED_EDGE('',*,*,#16924,.T.);
#24048=ORIENTED_EDGE('',*,*,#16920,.F.);
#24049=ORIENTED_EDGE('',*,*,#16925,.T.);
#24050=ORIENTED_EDGE('',*,*,#16904,.T.);
#24051=ORIENTED_EDGE('',*,*,#16837,.T.);
#24052=ORIENTED_EDGE('',*,*,#16914,.F.);
#24053=ORIENTED_EDGE('',*,*,#16905,.F.);
#24054=ORIENTED_EDGE('',*,*,#16908,.F.);
#24055=ORIENTED_EDGE('',*,*,#16887,.F.);
#24056=ORIENTED_EDGE('',*,*,#16871,.F.);
#24057=ORIENTED_EDGE('',*,*,#16875,.F.);
#24058=ORIENTED_EDGE('',*,*,#16889,.F.);
#24059=ORIENTED_EDGE('',*,*,#16923,.F.);
#24060=ORIENTED_EDGE('',*,*,#16919,.F.);
#24061=ORIENTED_EDGE('',*,*,#16899,.F.);
#24062=ORIENTED_EDGE('',*,*,#16893,.F.);
#24063=ORIENTED_EDGE('',*,*,#16890,.F.);
#24064=ORIENTED_EDGE('',*,*,#16885,.F.);
#24065=ORIENTED_EDGE('',*,*,#16881,.F.);
#24066=ORIENTED_EDGE('',*,*,#16877,.F.);
#24067=ORIENTED_EDGE('',*,*,#16913,.F.);
#24068=ORIENTED_EDGE('',*,*,#16922,.F.);
#24069=ORIENTED_EDGE('',*,*,#16918,.F.);
#24070=ORIENTED_EDGE('',*,*,#16926,.T.);
#24071=ORIENTED_EDGE('',*,*,#16925,.F.);
#24072=ORIENTED_EDGE('',*,*,#16926,.F.);
#24073=ORIENTED_EDGE('',*,*,#16924,.F.);
#24074=ORIENTED_EDGE('',*,*,#16909,.F.);
#24075=ORIENTED_EDGE('',*,*,#16915,.F.);
#24076=ORIENTED_EDGE('',*,*,#16897,.F.);
#24077=ORIENTED_EDGE('',*,*,#16901,.F.);
#24078=ORIENTED_EDGE('',*,*,#16921,.F.);
#24079=ORIENTED_EDGE('',*,*,#16833,.F.);
#24080=ORIENTED_EDGE('',*,*,#16851,.F.);
#24081=ORIENTED_EDGE('',*,*,#16927,.T.);
#24082=ORIENTED_EDGE('',*,*,#16883,.F.);
#24083=ORIENTED_EDGE('',*,*,#16892,.F.);
#24084=ORIENTED_EDGE('',*,*,#16843,.T.);
#24085=ORIENTED_EDGE('',*,*,#16884,.F.);
#24086=ORIENTED_EDGE('',*,*,#16927,.F.);
#24087=ORIENTED_EDGE('',*,*,#16850,.F.);
#24088=ORIENTED_EDGE('',*,*,#16854,.F.);
#26758=PLANE('',#30239);
#26759=PLANE('',#30240);
#26760=PLANE('',#30241);
#26761=PLANE('',#30242);
#26762=PLANE('',#30243);
#26763=PLANE('',#30244);
#26764=PLANE('',#30245);
#26765=PLANE('',#30246);
#26766=PLANE('',#30247);
#26767=PLANE('',#30248);
#26768=PLANE('',#30249);
#26769=PLANE('',#30250);
#26770=PLANE('',#30251);
#26771=PLANE('',#30252);
#26772=PLANE('',#30253);
#26773=PLANE('',#30254);
#26774=PLANE('',#30255);
#26775=PLANE('',#30256);
#26776=PLANE('',#30257);
#26777=PLANE('',#30258);
#26778=PLANE('',#30259);
#26779=PLANE('',#30260);
#26780=PLANE('',#30261);
#26781=PLANE('',#30262);
#26782=PLANE('',#30263);
#26783=PLANE('',#30264);
#26784=PLANE('',#30265);
#26785=PLANE('',#30266);
#26786=PLANE('',#30267);
#26787=PLANE('',#30268);
#26788=PLANE('',#30269);
#26789=PLANE('',#30270);
#26790=PLANE('',#30271);
#26791=PLANE('',#30272);
#26792=PLANE('',#30273);
#26793=PLANE('',#30274);
#26794=PLANE('',#30275);
#26795=PLANE('',#30276);
#26796=PLANE('',#30277);
#26797=PLANE('',#30278);
#26798=PLANE('',#30279);
#26799=PLANE('',#30280);
#26800=PLANE('',#30281);
#26801=PLANE('',#30282);
#26802=PLANE('',#30283);
#28026=ADVANCED_FACE('',(#4118),#26758,.T.);
#28027=ADVANCED_FACE('',(#4119),#26759,.T.);
#28028=ADVANCED_FACE('',(#4120),#26760,.T.);
#28029=ADVANCED_FACE('',(#4121),#26761,.T.);
#28030=ADVANCED_FACE('',(#4122),#26762,.T.);
#28031=ADVANCED_FACE('',(#4123),#26763,.T.);
#28032=ADVANCED_FACE('',(#4124),#26764,.T.);
#28033=ADVANCED_FACE('',(#4125),#26765,.T.);
#28034=ADVANCED_FACE('',(#4126),#26766,.T.);
#28035=ADVANCED_FACE('',(#4127),#26767,.T.);
#28036=ADVANCED_FACE('',(#4128),#26768,.T.);
#28037=ADVANCED_FACE('',(#4129),#26769,.T.);
#28038=ADVANCED_FACE('',(#4130),#26770,.T.);
#28039=ADVANCED_FACE('',(#4131),#26771,.T.);
#28040=ADVANCED_FACE('',(#4132),#26772,.T.);
#28041=ADVANCED_FACE('',(#4133),#26773,.T.);
#28042=ADVANCED_FACE('',(#4134),#26774,.T.);
#28043=ADVANCED_FACE('',(#4135),#26775,.T.);
#28044=ADVANCED_FACE('',(#4136),#26776,.T.);
#28045=ADVANCED_FACE('',(#4137),#26777,.T.);
#28046=ADVANCED_FACE('',(#4138),#26778,.T.);
#28047=ADVANCED_FACE('',(#4139),#26779,.T.);
#28048=ADVANCED_FACE('',(#4140),#26780,.T.);
#28049=ADVANCED_FACE('',(#4141),#26781,.T.);
#28050=ADVANCED_FACE('',(#4142),#26782,.T.);
#28051=ADVANCED_FACE('',(#4143),#26783,.T.);
#28052=ADVANCED_FACE('',(#4144),#26784,.T.);
#28053=ADVANCED_FACE('',(#4145),#26785,.T.);
#28054=ADVANCED_FACE('',(#4146),#26786,.T.);
#28055=ADVANCED_FACE('',(#4147),#26787,.T.);
#28056=ADVANCED_FACE('',(#4148),#26788,.T.);
#28057=ADVANCED_FACE('',(#4149),#26789,.T.);
#28058=ADVANCED_FACE('',(#4150),#26790,.T.);
#28059=ADVANCED_FACE('',(#4151),#26791,.T.);
#28060=ADVANCED_FACE('',(#4152),#26792,.T.);
#28061=ADVANCED_FACE('',(#4153),#26793,.T.);
#28062=ADVANCED_FACE('',(#4154),#26794,.T.);
#28063=ADVANCED_FACE('',(#4155),#26795,.T.);
#28064=ADVANCED_FACE('',(#4156),#26796,.T.);
#28065=ADVANCED_FACE('',(#4157),#26797,.F.);
#28066=ADVANCED_FACE('',(#4158),#26798,.F.);
#28067=ADVANCED_FACE('',(#4159),#26799,.F.);
#28068=ADVANCED_FACE('',(#4160),#26800,.T.);
#28069=ADVANCED_FACE('',(#4161),#26801,.T.);
#28070=ADVANCED_FACE('',(#4162),#26802,.T.);
#28472=CLOSED_SHELL('',(#28026,#28027,#28028,#28029,#28030,#28031,#28032,
#28033,#28034,#28035,#28036,#28037,#28038,#28039,#28040,#28041,#28042,#28043,
#28044,#28045,#28046,#28047,#28048,#28049,#28050,#28051,#28052,#28053,#28054,
#28055,#28056,#28057,#28058,#28059,#28060,#28061,#28062,#28063,#28064,#28065,
#28066,#28067,#28068,#28069,#28070));
#30238=AXIS2_PLACEMENT_3D('',#58854,#35921,#35922);
#30239=AXIS2_PLACEMENT_3D('',#58855,#35923,#35924);
#30240=AXIS2_PLACEMENT_3D('',#58868,#35931,#35932);
#30241=AXIS2_PLACEMENT_3D('',#58874,#35936,#35937);
#30242=AXIS2_PLACEMENT_3D('',#58882,#35942,#35943);
#30243=AXIS2_PLACEMENT_3D('',#58890,#35948,#35949);
#30244=AXIS2_PLACEMENT_3D('',#58906,#35958,#35959);
#30245=AXIS2_PLACEMENT_3D('',#58910,#35962,#35963);
#30246=AXIS2_PLACEMENT_3D('',#58918,#35968,#35969);
#30247=AXIS2_PLACEMENT_3D('',#58924,#35973,#35974);
#30248=AXIS2_PLACEMENT_3D('',#58930,#35978,#35979);
#30249=AXIS2_PLACEMENT_3D('',#58943,#35986,#35987);
#30250=AXIS2_PLACEMENT_3D('',#58949,#35991,#35992);
#30251=AXIS2_PLACEMENT_3D('',#58954,#35996,#35997);
#30252=AXIS2_PLACEMENT_3D('',#58956,#35999,#36000);
#30253=AXIS2_PLACEMENT_3D('',#58960,#36003,#36004);
#30254=AXIS2_PLACEMENT_3D('',#58968,#36009,#36010);
#30255=AXIS2_PLACEMENT_3D('',#58974,#36014,#36015);
#30256=AXIS2_PLACEMENT_3D('',#58978,#36018,#36019);
#30257=AXIS2_PLACEMENT_3D('',#58982,#36022,#36023);
#30258=AXIS2_PLACEMENT_3D('',#58985,#36026,#36027);
#30259=AXIS2_PLACEMENT_3D('',#58993,#36032,#36033);
#30260=AXIS2_PLACEMENT_3D('',#58999,#36037,#36038);
#30261=AXIS2_PLACEMENT_3D('',#59000,#36039,#36040);
#30262=AXIS2_PLACEMENT_3D('',#59005,#36044,#36045);
#30263=AXIS2_PLACEMENT_3D('',#59011,#36049,#36050);
#30264=AXIS2_PLACEMENT_3D('',#59017,#36054,#36055);
#30265=AXIS2_PLACEMENT_3D('',#59023,#36059,#36060);
#30266=AXIS2_PLACEMENT_3D('',#59029,#36064,#36065);
#30267=AXIS2_PLACEMENT_3D('',#59031,#36067,#36068);
#30268=AXIS2_PLACEMENT_3D('',#59035,#36071,#36072);
#30269=AXIS2_PLACEMENT_3D('',#59038,#36075,#36076);
#30270=AXIS2_PLACEMENT_3D('',#59044,#36080,#36081);
#30271=AXIS2_PLACEMENT_3D('',#59048,#36084,#36085);
#30272=AXIS2_PLACEMENT_3D('',#59050,#36087,#36088);
#30273=AXIS2_PLACEMENT_3D('',#59054,#36091,#36092);
#30274=AXIS2_PLACEMENT_3D('',#59060,#36096,#36097);
#30275=AXIS2_PLACEMENT_3D('',#59063,#36100,#36101);
#30276=AXIS2_PLACEMENT_3D('',#59066,#36104,#36105);
#30277=AXIS2_PLACEMENT_3D('',#59068,#36107,#36108);
#30278=AXIS2_PLACEMENT_3D('',#59069,#36109,#36110);
#30279=AXIS2_PLACEMENT_3D('',#59070,#36111,#36112);
#30280=AXIS2_PLACEMENT_3D('',#59072,#36114,#36115);
#30281=AXIS2_PLACEMENT_3D('',#59073,#36116,#36117);
#30282=AXIS2_PLACEMENT_3D('',#59074,#36118,#36119);
#30283=AXIS2_PLACEMENT_3D('',#59076,#36121,#36122);
#35921=DIRECTION('axis',(0.,0.,1.));
#35922=DIRECTION('refdir',(1.,0.,0.));
#35923=DIRECTION('center_axis',(0.,0.707106781186522,-0.707106781186573));
#35924=DIRECTION('ref_axis',(-1.,0.,0.));
#35925=DIRECTION('',(0.577350269189634,0.577350269189642,0.577350269189601));
#35926=DIRECTION('',(1.,0.,0.));
#35927=DIRECTION('',(0.577350269189633,-0.577350269189643,-0.577350269189602));
#35928=DIRECTION('',(-0.577350269189594,-0.577350269189662,-0.577350269189621));
#35929=DIRECTION('',(-1.,0.,0.));
#35930=DIRECTION('',(-0.577350269189598,0.57735026918966,0.577350269189619));
#35931=DIRECTION('center_axis',(0.,0.,-1.));
#35932=DIRECTION('ref_axis',(-1.,0.,0.));
#35933=DIRECTION('',(0.,1.,0.));
#35934=DIRECTION('',(1.,0.,0.));
#35935=DIRECTION('',(0.,-1.,0.));
#35936=DIRECTION('center_axis',(0.707106781186564,0.,-0.707106781186531));
#35937=DIRECTION('ref_axis',(-0.707106781186531,0.,-0.707106781186564));
#35938=DIRECTION('',(-0.577350269189613,0.577350269189624,-0.577350269189641));
#35939=DIRECTION('',(0.,-1.,0.));
#35940=DIRECTION('',(0.577350269189613,0.577350269189624,0.577350269189641));
#35941=DIRECTION('',(0.577350269189594,-0.577350269189662,0.577350269189621));
#35942=DIRECTION('center_axis',(0.707106781186554,0.707106781186541,0.));
#35943=DIRECTION('ref_axis',(0.,0.,-1.));
#35944=DIRECTION('',(0.,0.,1.));
#35945=DIRECTION('',(0.577350269189633,-0.577350269189643,0.577350269189602));
#35946=DIRECTION('',(0.577350269189615,-0.577350269189626,-0.577350269189636));
#35947=DIRECTION('',(0.,0.,-1.));
#35948=DIRECTION('center_axis',(0.,1.,0.));
#35949=DIRECTION('ref_axis',(0.,0.,1.));
#35950=DIRECTION('',(0.,0.,-1.));
#35951=DIRECTION('',(-0.70710678118655,0.,-0.707106781186545));
#35952=DIRECTION('',(0.70710678118655,0.,-0.707106781186545));
#35953=DIRECTION('',(0.,0.,-1.));
#35954=DIRECTION('',(-1.,0.,0.));
#35955=DIRECTION('',(-0.707106781186548,0.,0.707106781186548));
#35956=DIRECTION('',(-0.707106781186548,0.,-0.707106781186548));
#35957=DIRECTION('',(-1.,0.,0.));
#35958=DIRECTION('center_axis',(1.,0.,0.));
#35959=DIRECTION('ref_axis',(0.,0.,-1.));
#35960=DIRECTION('',(0.,1.,0.));
#35961=DIRECTION('',(0.,0.,1.));
#35962=DIRECTION('center_axis',(-0.499999999999988,0.707106781186564,0.499999999999988));
#35963=DIRECTION('ref_axis',(0.707106781186548,0.,0.707106781186548));
#35964=DIRECTION('',(0.281084637714915,0.678598344545852,-0.678598344545803));
#35965=DIRECTION('',(0.,0.577350269189608,-0.816496580927739));
#35966=DIRECTION('',(0.707106781186548,0.,0.707106781186548));
#35967=DIRECTION('',(0.862856209461028,0.357406744336628,0.357406744336531));
#35968=DIRECTION('center_axis',(0.,0.707106781186522,0.707106781186573));
#35969=DIRECTION('ref_axis',(1.,0.,0.));
#35970=DIRECTION('',(-0.862856209461047,0.357406744336575,-0.357406744336539));
#35971=DIRECTION('',(1.,0.,0.));
#35972=DIRECTION('',(0.577350269189598,0.57735026918966,-0.577350269189619));
#35973=DIRECTION('center_axis',(-0.382683432365029,0.,0.923879532511312));
#35974=DIRECTION('ref_axis',(0.923879532511312,0.,0.382683432365029));
#35975=DIRECTION('',(0.,-1.,0.));
#35976=DIRECTION('',(0.923879532511312,0.,0.382683432365029));
#35977=DIRECTION('',(0.,1.,0.));
#35978=DIRECTION('center_axis',(0.382683432365106,0.,0.92387953251128));
#35979=DIRECTION('ref_axis',(0.92387953251128,0.,-0.382683432365106));
#35980=DIRECTION('',(-0.862856209460998,-0.357406744336628,0.357406744336603));
#35981=DIRECTION('',(0.,-1.,0.));
#35982=DIRECTION('',(0.862856209460998,-0.357406744336628,-0.357406744336603));
#35983=DIRECTION('',(0.86285620946102,0.357406744336566,-0.357406744336612));
#35984=DIRECTION('',(0.,1.,0.));
#35985=DIRECTION('',(-0.86285620946102,0.357406744336566,0.357406744336612));
#35986=DIRECTION('center_axis',(0.,0.,1.));
#35987=DIRECTION('ref_axis',(1.,0.,0.));
#35988=DIRECTION('',(1.,0.,0.));
#35989=DIRECTION('',(0.,1.,0.));
#35990=DIRECTION('',(-1.,0.,0.));
#35991=DIRECTION('center_axis',(0.,0.707106781186522,0.707106781186573));
#35992=DIRECTION('ref_axis',(1.,0.,0.));
#35993=DIRECTION('',(0.281084637714926,-0.678598344545849,0.678598344545801));
#35994=DIRECTION('',(-0.577350269189634,-0.577350269189642,0.577350269189601));
#35995=DIRECTION('',(0.577350269189597,-0.577350269189661,0.57735026918962));
#35996=DIRECTION('center_axis',(0.499999999999988,0.707106781186564,0.499999999999988));
#35997=DIRECTION('ref_axis',(0.707106781186548,0.,-0.707106781186548));
#35998=DIRECTION('',(0.707106781186548,0.,-0.707106781186548));
#35999=DIRECTION('center_axis',(0.707106781186548,0.,0.707106781186548));
#36000=DIRECTION('ref_axis',(0.707106781186548,0.,-0.707106781186548));
#36001=DIRECTION('',(-0.707106781186548,0.,0.707106781186548));
#36002=DIRECTION('',(0.,1.,0.));
#36003=DIRECTION('center_axis',(-0.707106781186561,0.,0.707106781186534));
#36004=DIRECTION('ref_axis',(0.707106781186534,0.,0.707106781186561));
#36005=DIRECTION('',(0.577350269189616,0.577350269189624,0.577350269189638));
#36006=DIRECTION('',(0.,-1.,0.));
#36007=DIRECTION('',(-0.577350269189616,0.577350269189624,-0.577350269189638));
#36008=DIRECTION('',(-0.577350269189597,-0.577350269189661,-0.57735026918962));
#36009=DIRECTION('center_axis',(0.,-0.707106781186522,0.707106781186573));
#36010=DIRECTION('ref_axis',(1.,0.,0.));
#36011=DIRECTION('',(0.577350269189634,-0.577350269189642,-0.577350269189601));
#36012=DIRECTION('',(1.,0.,0.));
#36013=DIRECTION('',(0.281084637714926,0.678598344545849,0.678598344545801));
#36014=DIRECTION('center_axis',(0.499999999999988,-0.707106781186564,0.499999999999988));
#36015=DIRECTION('ref_axis',(0.707106781186548,0.,-0.707106781186548));
#36016=DIRECTION('',(0.707106781186548,0.,-0.707106781186548));
#36017=DIRECTION('',(-1.02558009940453E-14,0.577350269189613,0.816496580927735));
#36018=DIRECTION('center_axis',(-0.313549377219788,-0.573302186256024,0.756975158957774));
#36019=DIRECTION('ref_axis',(0.923879532511309,0.,0.382683432365036));
#36020=DIRECTION('',(-0.732537816328754,0.653281482438167,0.191341716182569));
#36021=DIRECTION('',(-0.38268343236507,-0.653281482438217,-0.653281482438171));
#36022=DIRECTION('center_axis',(-0.499999999999988,-0.707106781186564,0.499999999999988));
#36023=DIRECTION('ref_axis',(0.707106781186548,0.,0.707106781186548));
#36024=DIRECTION('',(0.707106781186548,0.,0.707106781186548));
#36025=DIRECTION('',(-0.707106781186548,0.,-0.707106781186548));
#36026=DIRECTION('center_axis',(0.,-0.707106781186522,0.707106781186573));
#36027=DIRECTION('ref_axis',(1.,0.,0.));
#36028=DIRECTION('',(-0.577350269189598,0.57735026918966,0.577350269189619));
#36029=DIRECTION('',(-1.,0.,0.));
#36030=DIRECTION('',(1.,0.,0.));
#36031=DIRECTION('',(0.577350269189633,0.577350269189643,0.577350269189602));
#36032=DIRECTION('center_axis',(-0.707106781186552,-0.707106781186543,0.));
#36033=DIRECTION('ref_axis',(0.,0.,1.));
#36034=DIRECTION('',(0.,0.,-1.));
#36035=DIRECTION('',(0.653281482438191,-0.6532814824382,-0.382683432365065));
#36036=DIRECTION('',(0.,0.,1.));
#36037=DIRECTION('center_axis',(-0.707106781186548,0.,0.707106781186548));
#36038=DIRECTION('ref_axis',(0.707106781186548,0.,0.707106781186548));
#36039=DIRECTION('center_axis',(0.707106781186554,-0.707106781186541,0.));
#36040=DIRECTION('ref_axis',(0.,0.,-1.));
#36041=DIRECTION('',(0.,0.,-1.));
#36042=DIRECTION('',(0.577350269189633,0.577350269189643,-0.577350269189602));
#36043=DIRECTION('',(-0.577350269189615,-0.577350269189626,0.577350269189636));
#36044=DIRECTION('center_axis',(0.,-0.707106781186522,-0.707106781186573));
#36045=DIRECTION('ref_axis',(-1.,0.,0.));
#36046=DIRECTION('',(-1.,0.,0.));
#36047=DIRECTION('',(-0.577350269189634,0.577350269189642,-0.577350269189601));
#36048=DIRECTION('',(0.577350269189598,0.57735026918966,-0.577350269189619));
#36049=DIRECTION('center_axis',(-0.70710678118656,0.,-0.707106781186535));
#36050=DIRECTION('ref_axis',(-0.707106781186535,0.,0.70710678118656));
#36051=DIRECTION('',(0.577350269189616,-0.577350269189624,-0.577350269189637));
#36052=DIRECTION('',(0.,1.,0.));
#36053=DIRECTION('',(-0.577350269189616,-0.577350269189624,0.577350269189637));
#36054=DIRECTION('center_axis',(-0.707106781186552,-0.707106781186543,0.));
#36055=DIRECTION('ref_axis',(0.,0.,1.));
#36056=DIRECTION('',(0.,0.,1.));
#36057=DIRECTION('',(-0.653281482438214,0.653281482438223,-0.382683432364986));
#36058=DIRECTION('',(0.,0.,-1.));
#36059=DIRECTION('center_axis',(-0.756975158957757,0.573302186256023,-0.31354937721983));
#36060=DIRECTION('ref_axis',(-0.382683432365087,0.,0.923879532511288));
#36061=DIRECTION('',(0.382683432365099,0.,-0.923879532511283));
#36062=DIRECTION('',(-0.653281482438191,-0.6532814824382,0.382683432365065));
#36063=DIRECTION('',(0.191341716182552,0.653281482438187,0.732537816328741));
#36064=DIRECTION('center_axis',(-0.707106781186552,0.707106781186543,0.));
#36065=DIRECTION('ref_axis',(0.,0.,1.));
#36066=DIRECTION('',(0.,0.,1.));
#36067=DIRECTION('center_axis',(-0.756975158957749,-0.573302186256029,-0.313549377219838));
#36068=DIRECTION('ref_axis',(-0.382683432365099,0.,0.923879532511283));
#36069=DIRECTION('',(-0.382683432365099,0.,0.923879532511283));
#36070=DIRECTION('',(-0.191341716182552,0.653281482438187,-0.732537816328741));
#36071=DIRECTION('center_axis',(-0.923879532511283,0.,-0.382683432365099));
#36072=DIRECTION('ref_axis',(-0.382683432365099,0.,0.923879532511283));
#36073=DIRECTION('',(0.,1.,0.));
#36074=DIRECTION('',(0.,-1.,0.));
#36075=DIRECTION('center_axis',(-0.756975158957738,0.573302186256039,0.313549377219846));
#36076=DIRECTION('ref_axis',(0.382683432365112,0.,0.923879532511278));
#36077=DIRECTION('',(-0.382683432365099,0.,-0.923879532511283));
#36078=DIRECTION('',(-0.191341716182505,-0.653281482438147,0.732537816328789));
#36079=DIRECTION('',(0.653281482438214,0.653281482438223,0.382683432364986));
#36080=DIRECTION('center_axis',(-0.499999999999985,0.707106781186566,0.499999999999989));
#36081=DIRECTION('ref_axis',(0.70710678118655,0.,0.707106781186545));
#36082=DIRECTION('',(0.70710678118655,0.,0.707106781186545));
#36083=DIRECTION('',(0.816496580927738,0.577350269189609,0.));
#36084=DIRECTION('center_axis',(-0.707106781186552,0.707106781186543,0.));
#36085=DIRECTION('ref_axis',(0.,0.,1.));
#36086=DIRECTION('',(0.,0.,1.));
#36087=DIRECTION('center_axis',(-0.756975158957738,-0.573302186256037,0.31354937721985));
#36088=DIRECTION('ref_axis',(0.382683432365116,0.,0.923879532511276));
#36089=DIRECTION('',(0.382683432365099,0.,0.923879532511283));
#36090=DIRECTION('',(0.1913417161825,-0.653281482438148,-0.73253781632879));
#36091=DIRECTION('center_axis',(-0.499999999999985,-0.707106781186566,0.499999999999989));
#36092=DIRECTION('ref_axis',(0.70710678118655,0.,0.707106781186545));
#36093=DIRECTION('',(-0.70710678118655,0.,-0.707106781186545));
#36094=DIRECTION('',(0.70710678118655,0.,0.707106781186545));
#36095=DIRECTION('',(-0.816496580927738,0.577350269189609,0.));
#36096=DIRECTION('center_axis',(-0.923879532511283,0.,0.382683432365099));
#36097=DIRECTION('ref_axis',(0.382683432365099,0.,0.923879532511283));
#36098=DIRECTION('',(0.,-1.,0.));
#36099=DIRECTION('',(0.,1.,0.));
#36100=DIRECTION('center_axis',(-0.499999999999991,-0.707106781186558,-0.499999999999994));
#36101=DIRECTION('ref_axis',(-0.70710678118655,0.,0.707106781186545));
#36102=DIRECTION('',(-0.70710678118655,0.,0.707106781186545));
#36103=DIRECTION('',(0.70710678118655,0.,-0.707106781186545));
#36104=DIRECTION('center_axis',(-0.499999999999991,0.707106781186558,-0.499999999999994));
#36105=DIRECTION('ref_axis',(-0.70710678118655,0.,0.707106781186545));
#36106=DIRECTION('',(-0.70710678118655,0.,0.707106781186545));
#36107=DIRECTION('center_axis',(-1.,0.,0.));
#36108=DIRECTION('ref_axis',(0.,0.,1.));
#36109=DIRECTION('center_axis',(0.,1.,0.));
#36110=DIRECTION('ref_axis',(1.,0.,0.));
#36111=DIRECTION('center_axis',(0.707106781186545,0.,-0.70710678118655));
#36112=DIRECTION('ref_axis',(-0.70710678118655,0.,-0.707106781186545));
#36113=DIRECTION('',(0.,1.,0.));
#36114=DIRECTION('center_axis',(0.707106781186545,0.,0.70710678118655));
#36115=DIRECTION('ref_axis',(0.70710678118655,0.,-0.707106781186545));
#36116=DIRECTION('center_axis',(-1.,0.,0.));
#36117=DIRECTION('ref_axis',(0.,0.,1.));
#36118=DIRECTION('center_axis',(0.70710678118656,0.,0.707106781186535));
#36119=DIRECTION('ref_axis',(0.707106781186535,0.,-0.70710678118656));
#36120=DIRECTION('',(0.,-1.,0.));
#36121=DIRECTION('center_axis',(0.,0.,1.));
#36122=DIRECTION('ref_axis',(1.,0.,0.));
#58854=CARTESIAN_POINT('',(0.,0.,0.));
#58855=CARTESIAN_POINT('Origin',(7.25,9.95,86.05));
#58856=CARTESIAN_POINT('',(0.575000000000009,9.975,86.075));
#58857=CARTESIAN_POINT('',(0.6,10.,86.1));
#58858=CARTESIAN_POINT('',(1.82500000000003,11.225,87.325));
#58859=CARTESIAN_POINT('',(9.4,10.,86.1));
#58860=CARTESIAN_POINT('',(7.25,10.,86.1));
#58861=CARTESIAN_POINT('',(9.425,9.975,86.075));
#58862=CARTESIAN_POINT('',(8.59166666666667,10.8083333333333,86.9083333333333));
#58863=CARTESIAN_POINT('',(9.35,9.9,86.));
#58864=CARTESIAN_POINT('',(5.72500000000001,6.27499999999958,82.3749999999998));
#58865=CARTESIAN_POINT('',(0.65,9.9,86.));
#58866=CARTESIAN_POINT('',(7.25,9.9,86.));
#58867=CARTESIAN_POINT('',(5.02499999999994,5.5249999999996,81.6249999999999));
#58868=CARTESIAN_POINT('Origin',(9.5,-10.,86.));
#58869=CARTESIAN_POINT('',(9.35,-9.9,86.));
#58870=CARTESIAN_POINT('',(9.35,-10.,86.));
#58871=CARTESIAN_POINT('',(0.65,-9.9,86.));
#58872=CARTESIAN_POINT('',(7.25,-9.9,86.));
#58873=CARTESIAN_POINT('',(0.65,-10.,86.));
#58874=CARTESIAN_POINT('Origin',(9.425,-10.,86.075));
#58875=CARTESIAN_POINT('',(9.5,9.9,86.15));
#58876=CARTESIAN_POINT('',(13.2499999999999,6.15000000000002,89.9000000000001));
#58877=CARTESIAN_POINT('',(9.5,-9.9,86.15));
#58878=CARTESIAN_POINT('',(9.5,-10.,86.15));
#58879=CARTESIAN_POINT('',(9.425,-9.975,86.075));
#58880=CARTESIAN_POINT('',(9.91666666666667,-9.48333333333333,86.5666666666667));
#58881=CARTESIAN_POINT('',(9.05833333333337,-9.60833333333333,85.7083333333334));
#58882=CARTESIAN_POINT('Origin',(9.45,9.95,89.));
#58883=CARTESIAN_POINT('',(9.4,10.,89.9));
#58884=CARTESIAN_POINT('',(9.4,10.,89.));
#58885=CARTESIAN_POINT('',(9.425,9.975,89.925));
#58886=CARTESIAN_POINT('',(8.67499999999999,10.725,89.175));
#58887=CARTESIAN_POINT('',(9.5,9.9,89.85));
#58888=CARTESIAN_POINT('',(12.9166666666666,6.48333333333333,86.4333333333333));
#58889=CARTESIAN_POINT('',(9.5,9.9,89.));
#58890=CARTESIAN_POINT('Origin',(5.,10.,88.));
#58891=CARTESIAN_POINT('',(0.6,10.,87.1585786437627));
#58892=CARTESIAN_POINT('',(0.6,10.,87.));
#58893=CARTESIAN_POINT('',(1.44142135623732,10.,88.));
#58894=CARTESIAN_POINT('',(2.29571067811867,10.,88.8542893218813));
#58895=CARTESIAN_POINT('',(0.600000000000003,10.,88.8414213562373));
#58896=CARTESIAN_POINT('',(1.87071067811866,10.,87.5707106781187));
#58897=CARTESIAN_POINT('',(0.6,10.,89.9));
#58898=CARTESIAN_POINT('',(0.6,10.,87.));
#58899=CARTESIAN_POINT('',(3.45857864376267,10.,89.9));
#58900=CARTESIAN_POINT('',(2.75,10.,89.9));
#58901=CARTESIAN_POINT('',(5.,10.,88.3585786437627));
#58902=CARTESIAN_POINT('',(4.30428932188134,10.,89.0542893218813));
#58903=CARTESIAN_POINT('',(6.54142135623733,10.,89.9));
#58904=CARTESIAN_POINT('',(4.94571067811866,10.,88.3042893218813));
#58905=CARTESIAN_POINT('',(5.75,10.,89.9));
#58906=CARTESIAN_POINT('Origin',(9.5,-10.,90.));
#58907=CARTESIAN_POINT('',(9.5,-9.9,89.85));
#58908=CARTESIAN_POINT('',(9.5,-10.,89.85));
#58909=CARTESIAN_POINT('',(9.5,-9.9,89.));
#58910=CARTESIAN_POINT('Origin',(4.91035533905933,9.95,88.3396446609407));
#58911=CARTESIAN_POINT('',(6.51464466094067,9.93535533905933,89.9646446609407));
#58912=CARTESIAN_POINT('',(6.58023082636872,10.0936943491397,89.8063056508603));
#58913=CARTESIAN_POINT('',(5.,9.9,88.5));
#58914=CARTESIAN_POINT('',(5.,9.81548220313558,88.6195262145876));
#58915=CARTESIAN_POINT('',(6.42928932188135,9.9,89.9292893218814));
#58916=CARTESIAN_POINT('',(4.875,9.9,88.375));
#58917=CARTESIAN_POINT('',(2.59518361520288,8.31186141672156,88.3411507386033));
#58918=CARTESIAN_POINT('Origin',(5.75,9.95,89.95));
#58919=CARTESIAN_POINT('',(6.60000000000001,9.9,90.));
#58920=CARTESIAN_POINT('',(6.60000000000001,9.9,90.));
#58921=CARTESIAN_POINT('',(9.35,9.9,90.));
#58922=CARTESIAN_POINT('',(5.75,9.9,90.));
#58923=CARTESIAN_POINT('',(5.47500000000001,6.0249999999996,93.8750000000001));
#58924=CARTESIAN_POINT('Origin',(6.51464466094068,-10.,89.9646446609407));
#58925=CARTESIAN_POINT('',(6.42928932188135,-9.9,89.9292893218814));
#58926=CARTESIAN_POINT('',(6.42928932188135,-10.,89.9292893218814));
#58927=CARTESIAN_POINT('',(6.60000000000001,-9.9,90.));
#58928=CARTESIAN_POINT('',(6.42928932188135,-9.9,89.9292893218814));
#58929=CARTESIAN_POINT('',(6.60000000000001,-10.,90.));
#58930=CARTESIAN_POINT('Origin',(3.48535533905933,-10.,89.9646446609407));
#58931=CARTESIAN_POINT('',(3.48535533905932,9.93535533905932,89.9646446609407));
#58932=CARTESIAN_POINT('',(3.4,9.9,90.));
#58933=CARTESIAN_POINT('',(0.142189545817937,8.55057072623677,91.3494292737631));
#58934=CARTESIAN_POINT('',(3.4,-9.9,90.));
#58935=CARTESIAN_POINT('',(3.4,-10.,90.));
#58936=CARTESIAN_POINT('',(3.48535533905932,-9.93535533905932,89.9646446609407));
#58937=CARTESIAN_POINT('',(3.22609583235893,-9.82796653520985,90.0720334647902));
#58938=CARTESIAN_POINT('',(3.57071067811866,-9.9,89.9292893218813));
#58939=CARTESIAN_POINT('',(3.92606829818375,-9.75280605427642,89.7820953761578));
#58940=CARTESIAN_POINT('',(3.57071067811866,9.9,89.9292893218813));
#58941=CARTESIAN_POINT('',(3.57071067811866,-10.,89.9292893218813));
#58942=CARTESIAN_POINT('',(7.00997458472428,8.47541024530379,88.504699567185));
#58943=CARTESIAN_POINT('Origin',(0.5,-10.,90.));
#58944=CARTESIAN_POINT('',(0.65,9.9,90.));
#58945=CARTESIAN_POINT('',(2.75,9.9,90.));
#58946=CARTESIAN_POINT('',(0.65,-9.9,90.));
#58947=CARTESIAN_POINT('',(0.65,-10.,90.));
#58948=CARTESIAN_POINT('',(2.75,-9.9,90.));
#58949=CARTESIAN_POINT('Origin',(2.75,9.95,89.95));
#58950=CARTESIAN_POINT('',(3.45857864376267,10.,89.9));
#58951=CARTESIAN_POINT('',(0.575000000000003,9.975,89.925));
#58952=CARTESIAN_POINT('',(1.40833333333333,10.8083333333333,89.0916666666667));
#58953=CARTESIAN_POINT('',(4.27500000000001,6.2749999999996,93.6250000000001));
#58954=CARTESIAN_POINT('Origin',(4.33964466094067,9.95,89.0896446609407));
#58955=CARTESIAN_POINT('',(4.375,9.9,89.125));
#58956=CARTESIAN_POINT('Origin',(3.5,-10.,90.));
#58957=CARTESIAN_POINT('',(5.,-9.9,88.5));
#58958=CARTESIAN_POINT('',(4.375,-9.9,89.125));
#58959=CARTESIAN_POINT('',(5.,-10.,88.5));
#58960=CARTESIAN_POINT('Origin',(0.575,-10.,89.925));
#58961=CARTESIAN_POINT('',(0.5,9.9,89.85));
#58962=CARTESIAN_POINT('',(-3.24999999999993,6.15000000000002,86.0999999999999));
#58963=CARTESIAN_POINT('',(0.5,-9.9,89.85));
#58964=CARTESIAN_POINT('',(0.5,-10.,89.85));
#58965=CARTESIAN_POINT('',(0.575000000000006,-9.975,89.925));
#58966=CARTESIAN_POINT('',(0.0833333333333344,-9.48333333333333,89.4333333333333));
#58967=CARTESIAN_POINT('',(0.941666666666637,-9.60833333333333,90.2916666666666));
#58968=CARTESIAN_POINT('Origin',(2.75,-9.95,89.95));
#58969=CARTESIAN_POINT('',(0.6,-10.,89.9));
#58970=CARTESIAN_POINT('',(1.40833333333333,-10.8083333333333,89.0916666666667));
#58971=CARTESIAN_POINT('',(3.45857864376267,-10.,89.9));
#58972=CARTESIAN_POINT('',(2.75,-10.,89.9));
#58973=CARTESIAN_POINT('',(3.45857864376267,-10.,89.9));
#58974=CARTESIAN_POINT('Origin',(4.33964466094067,-9.95,89.0896446609407));
#58975=CARTESIAN_POINT('',(5.,-10.,88.3585786437627));
#58976=CARTESIAN_POINT('',(4.30428932188134,-10.,89.0542893218813));
#58977=CARTESIAN_POINT('',(5.,-10.,88.3585786437627));
#58978=CARTESIAN_POINT('Origin',(6.54142135623733,-10.,89.9));
#58979=CARTESIAN_POINT('',(6.54142135623733,-10.,89.9));
#58980=CARTESIAN_POINT('',(6.54142135623733,-10.,89.9));
#58981=CARTESIAN_POINT('',(6.60000000000001,-9.9,90.));
#58982=CARTESIAN_POINT('Origin',(4.91035533905933,-9.95,88.3396446609407));
#58983=CARTESIAN_POINT('',(4.94571067811866,-10.,88.3042893218813));
#58984=CARTESIAN_POINT('',(4.875,-9.9,88.375));
#58985=CARTESIAN_POINT('Origin',(5.75,-9.95,89.95));
#58986=CARTESIAN_POINT('',(9.425,-9.975,89.925));
#58987=CARTESIAN_POINT('',(9.35,-9.9,90.));
#58988=CARTESIAN_POINT('',(8.80833333333339,-9.35833333333333,90.5416666666666));
#58989=CARTESIAN_POINT('',(5.75,-9.9,90.));
#58990=CARTESIAN_POINT('',(9.4,-10.,89.9));
#58991=CARTESIAN_POINT('',(5.75,-10.,89.9));
#58992=CARTESIAN_POINT('',(8.67499999999999,-10.725,89.175));
#58993=CARTESIAN_POINT('Origin',(0.55,-9.95,87.));
#58994=CARTESIAN_POINT('',(0.5,-9.9,88.9));
#58995=CARTESIAN_POINT('',(0.5,-9.9,87.));
#58996=CARTESIAN_POINT('',(0.6,-10.,88.8414213562373));
#58997=CARTESIAN_POINT('',(0.5,-9.9,88.9));
#58998=CARTESIAN_POINT('',(0.6,-10.,87.));
#58999=CARTESIAN_POINT('Origin',(5.,-10.,88.5));
#59000=CARTESIAN_POINT('Origin',(9.45,-9.95,89.));
#59001=CARTESIAN_POINT('',(9.4,-10.,86.1));
#59002=CARTESIAN_POINT('',(9.4,-10.,89.));
#59003=CARTESIAN_POINT('',(8.59166666666667,-10.8083333333333,86.9083333333333));
#59004=CARTESIAN_POINT('',(9.58333333333333,-9.81666666666667,89.7666666666667));
#59005=CARTESIAN_POINT('Origin',(7.25,-9.95,86.05));
#59006=CARTESIAN_POINT('',(0.6,-10.,86.1));
#59007=CARTESIAN_POINT('',(7.25,-10.,86.1));
#59008=CARTESIAN_POINT('',(0.575000000000001,-9.975,86.075));
#59009=CARTESIAN_POINT('',(1.82500000000003,-11.225,87.325));
#59010=CARTESIAN_POINT('',(1.69166666666657,-8.85833333333333,84.9583333333334));
#59011=CARTESIAN_POINT('Origin',(0.575,-10.,86.075));
#59012=CARTESIAN_POINT('',(0.5,-9.9,86.15));
#59013=CARTESIAN_POINT('',(0.416666666666669,-9.81666666666667,86.2333333333333));
#59014=CARTESIAN_POINT('',(0.5,9.9,86.15));
#59015=CARTESIAN_POINT('',(0.5,-10.,86.15));
#59016=CARTESIAN_POINT('',(-2.9166666666666,6.48333333333335,89.5666666666667));
#59017=CARTESIAN_POINT('Origin',(0.55,-9.95,87.));
#59018=CARTESIAN_POINT('',(0.599999999999999,-10.,87.1585786437627));
#59019=CARTESIAN_POINT('',(0.6,-10.,87.));
#59020=CARTESIAN_POINT('',(0.5,-9.9,87.1));
#59021=CARTESIAN_POINT('',(0.6,-10.,87.1585786437627));
#59022=CARTESIAN_POINT('',(0.5,-9.9,87.));
#59023=CARTESIAN_POINT('Origin',(0.6,10.,88.8414213562373));
#59024=CARTESIAN_POINT('',(0.5,9.9,88.9));
#59025=CARTESIAN_POINT('',(0.570710678118656,9.9,88.7292893218813));
#59026=CARTESIAN_POINT('',(0.5,9.9,88.9));
#59027=CARTESIAN_POINT('',(0.6,10.,88.8414213562373));
#59028=CARTESIAN_POINT('',(0.570710678118656,9.9,88.7292893218813));
#59029=CARTESIAN_POINT('Origin',(0.55,9.95,87.));
#59030=CARTESIAN_POINT('',(0.5,9.9,87.));
#59031=CARTESIAN_POINT('Origin',(0.570710678118656,-9.9,88.7292893218813));
#59032=CARTESIAN_POINT('',(0.570710678118656,-9.9,88.7292893218813));
#59033=CARTESIAN_POINT('',(0.570710678118656,-9.9,88.7292893218813));
#59034=CARTESIAN_POINT('',(0.600000000000003,-10.,88.8414213562373));
#59035=CARTESIAN_POINT('Origin',(0.535355339059328,-10.,88.8146446609407));
#59036=CARTESIAN_POINT('',(0.5,-10.,88.9));
#59037=CARTESIAN_POINT('',(0.570710678118656,-10.,88.7292893218813));
#59038=CARTESIAN_POINT('Origin',(0.599999999999999,10.,87.1585786437627));
#59039=CARTESIAN_POINT('',(0.570710678118658,9.9,87.2707106781187));
#59040=CARTESIAN_POINT('',(0.5,9.9,87.1));
#59041=CARTESIAN_POINT('',(0.570710678118656,9.9,87.2707106781187));
#59042=CARTESIAN_POINT('',(0.599999999999999,10.,87.1585786437627));
#59043=CARTESIAN_POINT('',(0.5,9.9,87.1));
#59044=CARTESIAN_POINT('Origin',(2.26035533905934,9.95,88.8896446609407));
#59045=CARTESIAN_POINT('',(1.3,9.9,88.));
#59046=CARTESIAN_POINT('',(2.22500000000001,9.9,88.925));
#59047=CARTESIAN_POINT('',(1.3,9.9,88.));
#59048=CARTESIAN_POINT('Origin',(0.55,9.95,87.));
#59049=CARTESIAN_POINT('',(0.5,9.9,87.));
#59050=CARTESIAN_POINT('Origin',(0.6,-10.,87.1585786437627));
#59051=CARTESIAN_POINT('',(0.570710678118656,-9.9,87.2707106781187));
#59052=CARTESIAN_POINT('',(0.5,-9.9,87.1));
#59053=CARTESIAN_POINT('',(0.570710678118658,-9.9,87.2707106781187));
#59054=CARTESIAN_POINT('Origin',(2.26035533905934,-9.95,88.8896446609407));
#59055=CARTESIAN_POINT('',(1.3,-9.9,88.));
#59056=CARTESIAN_POINT('',(2.22500000000001,-9.9,88.925));
#59057=CARTESIAN_POINT('',(1.44142135623732,-10.,88.));
#59058=CARTESIAN_POINT('',(2.29571067811867,-10.,88.8542893218813));
#59059=CARTESIAN_POINT('',(1.44142135623732,-10.,88.));
#59060=CARTESIAN_POINT('Origin',(0.535355339059328,-10.,87.1853553390593));
#59061=CARTESIAN_POINT('',(0.5,-10.,87.1));
#59062=CARTESIAN_POINT('',(0.570710678118656,-10.,87.2707106781187));
#59063=CARTESIAN_POINT('Origin',(1.83535533905933,-9.95,87.5353553390593));
#59064=CARTESIAN_POINT('',(1.87071067811866,-10.,87.5707106781187));
#59065=CARTESIAN_POINT('',(1.8,-9.9,87.5));
#59066=CARTESIAN_POINT('Origin',(1.83535533905933,9.95,87.5353553390593));
#59067=CARTESIAN_POINT('',(1.8,9.9,87.5));
#59068=CARTESIAN_POINT('Origin',(0.5,-10.,86.));
#59069=CARTESIAN_POINT('Origin',(5.,-10.,88.));
#59070=CARTESIAN_POINT('Origin',(1.3,-10.,88.));
#59071=CARTESIAN_POINT('',(1.3,-10.,88.));
#59072=CARTESIAN_POINT('Origin',(0.45,-10.,88.85));
#59073=CARTESIAN_POINT('Origin',(0.5,-10.,86.));
#59074=CARTESIAN_POINT('Origin',(9.425,-10.,89.925));
#59075=CARTESIAN_POINT('',(9.35,-10.,90.));
#59076=CARTESIAN_POINT('Origin',(6.5,-10.,90.));
#71465=UNCERTAINTY_MEASURE_WITH_UNIT(LENGTH_MEASURE(0.001),#71493,
'DISTANCE_ACCURACY_VALUE',
'Maximum model space distance between geometric entities at asserted c
onnectivities');
#71471=UNCERTAINTY_MEASURE_WITH_UNIT(LENGTH_MEASURE(0.001),#71493,
'DISTANCE_ACCURACY_VALUE',
'Maximum model space distance between geometric entities at asserted c
onnectivities');
#71486=(
GEOMETRIC_REPRESENTATION_CONTEXT(3)
GLOBAL_UNCERTAINTY_ASSIGNED_CONTEXT((#71465))
GLOBAL_UNIT_ASSIGNED_CONTEXT((#71493,#71495,#71496))
REPRESENTATION_CONTEXT('','3D')
);
#71492=(
GEOMETRIC_REPRESENTATION_CONTEXT(3)
GLOBAL_UNCERTAINTY_ASSIGNED_CONTEXT((#71471))
GLOBAL_UNIT_ASSIGNED_CONTEXT((#71493,#71495,#71496))
REPRESENTATION_CONTEXT('','3D')
);
#71493=(
LENGTH_UNIT()
NAMED_UNIT(*)
SI_UNIT(.CENTI.,.METRE.)
);
#71495=(
NAMED_UNIT(*)
PLANE_ANGLE_UNIT()
SI_UNIT($,.RADIAN.)
);
#71496=(
NAMED_UNIT(*)
SI_UNIT($,.STERADIAN.)
SOLID_ANGLE_UNIT()
);
#71511=SHAPE_DEFINITION_REPRESENTATION(#71531,#71616);
#71531=PRODUCT_DEFINITION_SHAPE('',$,#71637);
#71616=SHAPE_REPRESENTATION('',(#30238),#71486);
#71622=PRODUCT_DEFINITION_CONTEXT('part definition',#71684,'design');
#71637=PRODUCT_DEFINITION('2026-10-19-03-23-09-453',
'16_Press_V-Block_200x90x40',#71657,#71622);
#71657=PRODUCT_DEFINITION_FORMATION('',$,#71700);
#71684=APPLICATION_CONTEXT(
'Core Data for Automotive Mechanical Design Process');
#71685=PRODUCT_CONTEXT('part definition',#71684,'mechanical');
#71700=PRODUCT('2026-10-19-03-23-09-453','16_Press_V-Block_200x90x40',$,
(#71685));
#71860=COLOUR_RGB('Dark Blue',0.08,0.2,0.34);
#71861=FILL_AREA_STYLE_COLOUR('',#71860);
#71862=FILL_AREA_STYLE('',(#71861));
#71863=SURFACE_STYLE_FILL_AREA(#71862);
#71864=SURFACE_SIDE_STYLE('',(#71863));
#71865=SURFACE_STYLE_USAGE(.BOTH.,#71864);
#71866=PRESENTATION_STYLE_ASSIGNMENT((#71865));
ENDSEC;
END-ISO-10303-21;
